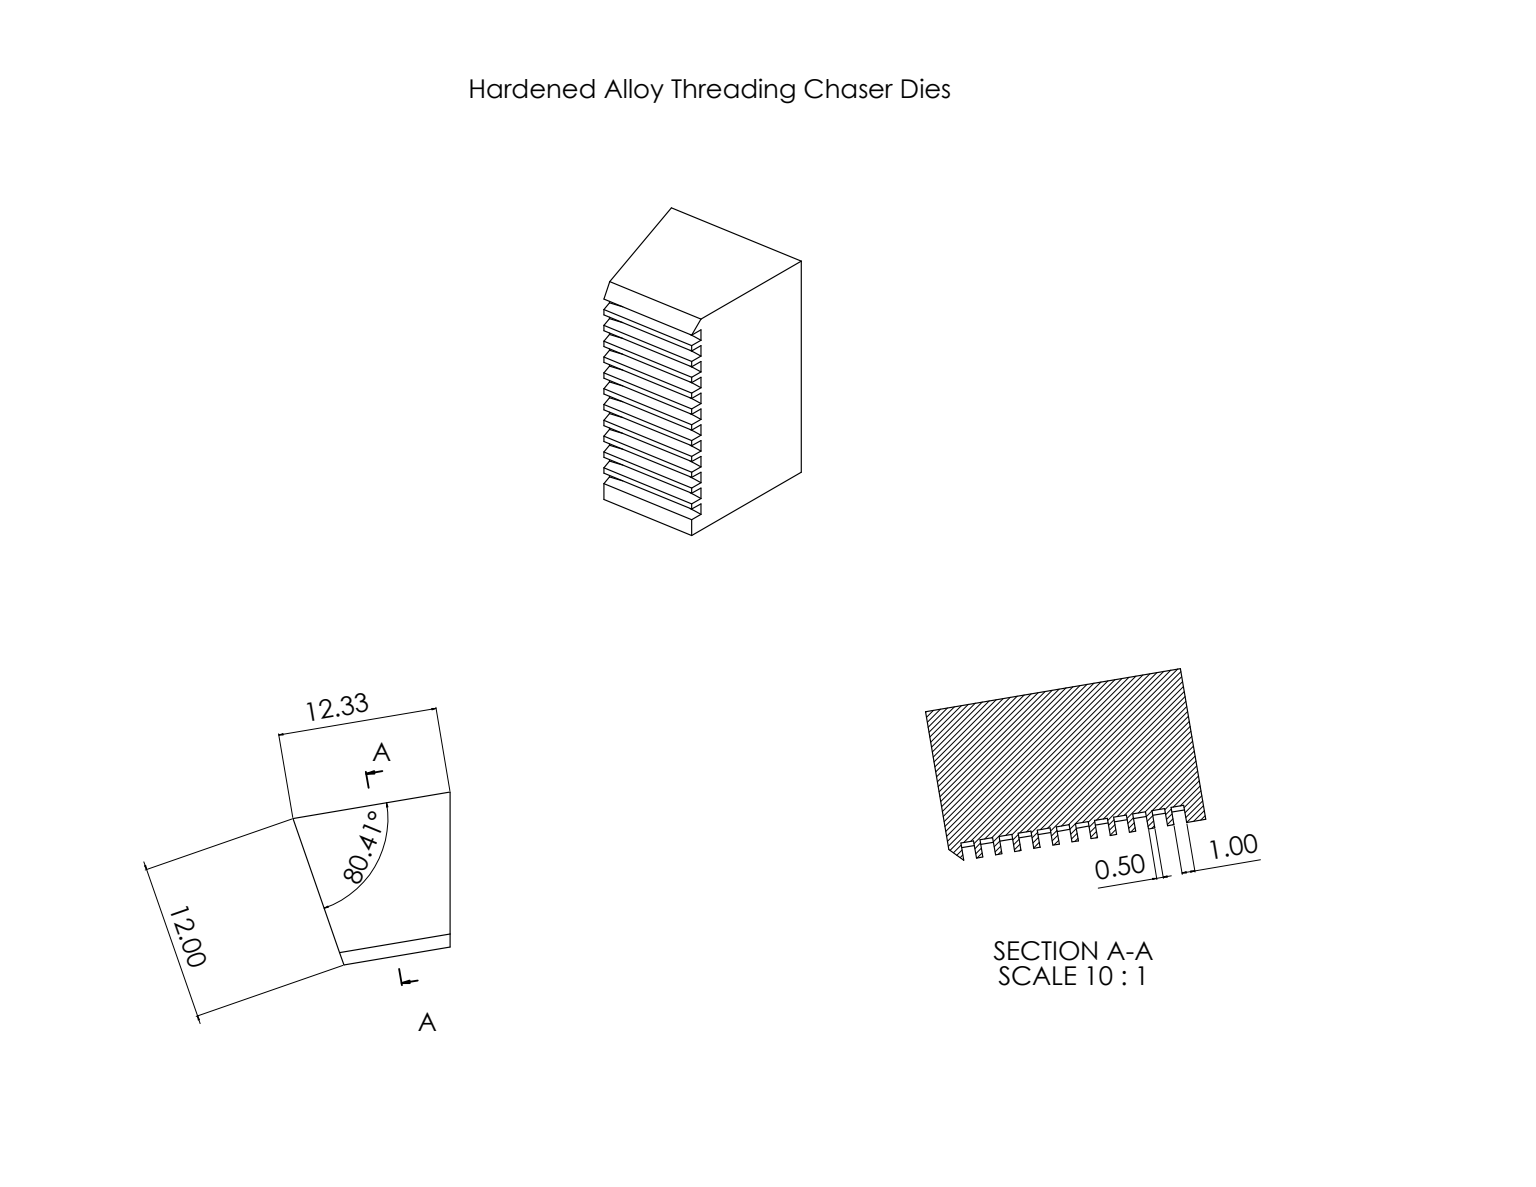
ISO-10303-21;
HEADER;
FILE_DESCRIPTION (('STEP AP214'),
    '1' );
FILE_NAME ('Hardened Alloy Threading Chaser Dies.step',
    '2026-10-19T14:05:14',
    ( '' ),
    ( '' ),
    'SwSTEP 2.0',
    'SolidWorks 2025',
    '' );
FILE_SCHEMA (( 'AUTOMOTIVE_DESIGN' ));
ENDSEC;

DATA;
#3=ORIENTED_EDGE ( 'NONE', *, *, #1774, .T. ) ;
#6=ORIENTED_EDGE ( 'NONE', *, *, #748, .T. ) ;
#8=LINE ( 'NONE', #7609, #8604 ) ;
#18=CARTESIAN_POINT ( 'NONE',  ( 1.030449557444946671E-26, 53.50000000000031264, -26.00000000000004974 ) ) ;
#24=ORIENTED_EDGE ( 'NONE', *, *, #464, .F. ) ;
#25=PRODUCT_DEFINITION_CONTEXT ( 'detailed design', #5808, 'design' ) ;
#30=FACE_OUTER_BOUND ( 'NONE', #6374, .T. ) ;
#38=CARTESIAN_POINT ( 'NONE',  ( 1.084683744678891232E-26, 59.63872771225970837, -25.64778813235487220 ) ) ;
#47=VECTOR ( 'NONE', #1280, 1000.000000000000000 ) ;
#49=VERTEX_POINT ( 'NONE', #7520 ) ;
#65=EDGE_LOOP ( 'NONE', ( #1698, #9286, #7170, #5423 ) ) ;
#70=CARTESIAN_POINT ( 'NONE',  ( 0.000000000000000000, 0.000000000000000000, 0.000000000000000000 ) ) ;
#75=DIRECTION ( 'NONE',  ( -1.735493991486225972E-29, 6.508102468073347395E-30, 1.000000000000000000 ) ) ;
#77=VERTEX_POINT ( 'NONE', #3810 ) ;
#83=CARTESIAN_POINT ( 'NONE',  ( 0.000000000000000000, 0.000000000000000000, 0.000000000000000000 ) ) ;
#90=AXIS2_PLACEMENT_3D ( 'NONE', #5171, #7481, #672 ) ;
#100=ORIENTED_EDGE ( 'NONE', *, *, #2687, .F. ) ;
#103=VECTOR ( 'NONE', #6274, 1000.000000000000341 ) ;
#104=CIRCLE ( 'NONE', #7815, 26.00000000000012790 ) ;
#107=EDGE_CURVE ( 'NONE', #2537, #9428, #3759, .T. ) ;
#110=CARTESIAN_POINT ( 'NONE',  ( 8.948640893600852668E-27, 42.50000000000020606, -25.00000000000000000 ) ) ;
#111=ORIENTED_EDGE ( 'NONE', *, *, #684, .T. ) ;
#114=ORIENTED_EDGE ( 'NONE', *, *, #8852, .F. ) ;
#117=AXIS2_PLACEMENT_3D ( 'NONE', #7294, #7143, #4982 ) ;
#119=CARTESIAN_POINT ( 'NONE',  ( -8.216777476527294510, 42.50000000000020606, -23.61111111111107519 ) ) ;
#125=CIRCLE ( 'NONE', #905, 26.00000000000000355 ) ;
#145=LINE ( 'NONE', #38, #7530 ) ;
#146=LINE ( 'NONE', #3335, #665 ) ;
#147=( LENGTH_UNIT ( ) NAMED_UNIT ( * ) SI_UNIT ( .MILLI., .METRE. ) );
#149=FACE_OUTER_BOUND ( 'NONE', #9484, .T. ) ;
#150=ADVANCED_FACE ( 'NONE', ( #6740 ), #686, .F. ) ;
#154=DIRECTION ( 'NONE',  ( 0.9860132971832693549, 1.788557213313974126E-28, -0.1666666666666657970 ) ) ;
#158=CARTESIAN_POINT ( 'NONE',  ( -8.216777476527294510, 50.00000000000032685, -23.61111111111111427 ) ) ;
#159=ORIENTED_EDGE ( 'NONE', *, *, #5056, .F. ) ;
#163=EDGE_CURVE ( 'NONE', #7794, #4048, #3844, .T. ) ;
#164=ADVANCED_FACE ( 'NONE', ( #5228 ), #5133, .F. ) ;
#185=VERTEX_POINT ( 'NONE', #9279 ) ;
#188=( GEOMETRIC_REPRESENTATION_CONTEXT ( 3 ) GLOBAL_UNCERTAINTY_ASSIGNED_CONTEXT ( ( #1496 ) ) GLOBAL_UNIT_ASSIGNED_CONTEXT ( ( #3676, #5943, #2174 ) ) REPRESENTATION_CONTEXT ( 'NONE', 'WORKASPACE' ) );
#195=ORIENTED_EDGE ( 'NONE', *, *, #1181, .F. ) ;
#214=CARTESIAN_POINT ( 'NONE',  ( 8.948640893600852668E-27, 42.50000000000020606, -25.00000000000000000 ) ) ;
#217=ADVANCED_FACE ( 'NONE', ( #8822 ), #7238, .F. ) ;
#226=EDGE_CURVE ( 'NONE', #987, #5419, #6349, .T. ) ;
#232=CARTESIAN_POINT ( 'NONE',  ( -8.545448575588375562, 56.00000000000030553, -24.55555555555558911 ) ) ;
#240=ORIENTED_EDGE ( 'NONE', *, *, #7837, .T. ) ;
#248=LINE ( 'NONE', #2485, #2906 ) ;
#250=AXIS2_PLACEMENT_3D ( 'NONE', #2833, #9708, #7388 ) ;
#255=EDGE_CURVE ( 'NONE', #1637, #4569, #2387, .T. ) ;
#260=DIRECTION ( 'NONE',  ( -1.735493991486225972E-29, 6.508102468073347395E-30, 1.000000000000000000 ) ) ;
#265=CARTESIAN_POINT ( 'NONE',  ( -8.216777476527294510, 56.50000000000029843, -23.61111111111111427 ) ) ;
#269=VERTEX_POINT ( 'NONE', #3889 ) ;
#274=VECTOR ( 'NONE', #1912, 1000.000000000000341 ) ;
#284=CARTESIAN_POINT ( 'NONE',  ( 9.318419442923201951E-27, 47.00000000000034106, -25.00000000000000000 ) ) ;
#302=CARTESIAN_POINT ( 'NONE',  ( 9.762153702110021092E-27, 45.50000000000019185, -25.00000000000000000 ) ) ;
#309=CARTESIAN_POINT ( 'NONE',  ( 9.219811829770575476E-27, 48.50000000000033396, -26.00000000000011369 ) ) ;
#318=ORIENTED_EDGE ( 'NONE', *, *, #9442, .F. ) ;
#319=AXIS2_PLACEMENT_3D ( 'NONE', #6643, #8980, #9669 ) ;
#321=ORIENTED_EDGE ( 'NONE', *, *, #7835, .T. ) ;
#336=VECTOR ( 'NONE', #2888, 1000.000000000000000 ) ;
#346=AXIS2_PLACEMENT_3D ( 'NONE', #4083, #2634, #9223 ) ;
#358=AXIS2_PLACEMENT_3D ( 'NONE', #6746, #9141, #8245 ) ;
#364=ORIENTED_EDGE ( 'NONE', *, *, #965, .F. ) ;
#369=ORIENTED_EDGE ( 'NONE', *, *, #9442, .T. ) ;
#375=CARTESIAN_POINT ( 'NONE',  ( 1.203012880462043003E-26, 59.00000000000029843, -25.00000000000000000 ) ) ;
#379=EDGE_LOOP ( 'NONE', ( #2512, #3295, #4858, #1225 ) ) ;
#382=FACE_OUTER_BOUND ( 'NONE', #3255, .T. ) ;
#393=DIRECTION ( 'NONE',  ( 1.735493991486225972E-29, -6.508102468073347395E-30, -1.000000000000000000 ) ) ;
#395=PLANE ( 'NONE',  #2897 ) ;
#408=ORIENTED_EDGE ( 'NONE', *, *, #8224, .T. ) ;
#445=FACE_OUTER_BOUND ( 'NONE', #6404, .T. ) ;
#451=DIRECTION ( 'NONE',  ( -1.735493991486225972E-29, 6.508102468073347395E-30, 1.000000000000000000 ) ) ;
#463=EDGE_CURVE ( 'NONE', #6976, #7794, #626, .T. ) ;
#464=EDGE_CURVE ( 'NONE', #7542, #9099, #8278, .T. ) ;
#467=LINE ( 'NONE', #608, #6068 ) ;
#468=EDGE_CURVE ( 'NONE', #5208, #1296, #1199, .T. ) ;
#473=ORIENTED_EDGE ( 'NONE', *, *, #8224, .F. ) ;
#478=VERTEX_POINT ( 'NONE', #8225 ) ;
#481=ORIENTED_EDGE ( 'NONE', *, *, #7790, .F. ) ;
#482=CARTESIAN_POINT ( 'NONE',  ( -8.216777476527274970, 48.50000000000033396, -23.61111111111111427 ) ) ;
#488=CARTESIAN_POINT ( 'NONE',  ( 1.555535097482682654E-26, 78.08723716182652197, -25.00000000000000000 ) ) ;
#495=PLANE ( 'NONE',  #7443 ) ;
#496=DIRECTION ( 'NONE',  ( -0.9860132971832694659, -1.788557213313974350E-28, 0.1666666666666658247 ) ) ;
#501=ORIENTED_EDGE ( 'NONE', *, *, #2623, .T. ) ;
#517=VERTEX_POINT ( 'NONE', #5126 ) ;
#518=EDGE_LOOP ( 'NONE', ( #1786, #1861, #2119, #8803 ) ) ;
#524=ADVANCED_FACE ( 'NONE', ( #4341 ), #7345, .F. ) ;
#530=ORIENTED_EDGE ( 'NONE', *, *, #3207, .T. ) ;
#532=VECTOR ( 'NONE', #9646, 1000.000000000000341 ) ;
#534=LINE ( 'NONE', #2734, #9462 ) ;
#544=CARTESIAN_POINT ( 'NONE',  ( 5.423418723394456162E-28, -2.066522830327504070E-28, -26.00000000000000355 ) ) ;
#545=DIRECTION ( 'NONE',  ( 1.735493991486223450E-29, 0.000000000000000000, -1.000000000000000000 ) ) ;
#553=EDGE_CURVE ( 'NONE', #1486, #2396, #9731, .T. ) ;
#554=ORIENTED_EDGE ( 'NONE', *, *, #4928, .F. ) ;
#571=AXIS2_PLACEMENT_3D ( 'NONE', #1883, #7968, #2471 ) ;
#574=EDGE_CURVE ( 'NONE', #9611, #2873, #3443, .T. ) ;
#578=CARTESIAN_POINT ( 'NONE',  ( 7.913260955498274673E-27, 41.50000000000020606, -26.00000000000017408 ) ) ;
#580=DIRECTION ( 'NONE',  ( -1.820952055660014662E-28, -1.000000000000000000, -7.038118388768679669E-30 ) ) ;
#586=EDGE_CURVE ( 'NONE', #9099, #2192, #627, .T. ) ;
#599=CARTESIAN_POINT ( 'NONE',  ( -8.216777476527274970, 47.50000000000033396, -23.61111111111111427 ) ) ;
#608=CARTESIAN_POINT ( 'NONE',  ( 1.040310318760209318E-26, 47.00000000000034106, -37.00000000000000711 ) ) ;
#611=ORIENTED_EDGE ( 'NONE', *, *, #2805, .F. ) ;
#615=CARTESIAN_POINT ( 'NONE',  ( 9.860761315262647568E-27, 50.00000000000032685, -24.09806918451531033 ) ) ;
#616=CARTESIAN_POINT ( 'NONE',  ( -8.216777476527274970, 78.08723716182652197, -23.61111111111111427 ) ) ;
#626=LINE ( 'NONE', #5323, #2764 ) ;
#627=LINE ( 'NONE', #6495, #5483 ) ;
#628=DIRECTION ( 'NONE',  ( 1.735493991486225692E-29, 0.000000000000000000, -1.000000000000000000 ) ) ;
#631=VECTOR ( 'NONE', #3107, 1000.000000000000000 ) ;
#643=ORIENTED_EDGE ( 'NONE', *, *, #1715, .F. ) ;
#647=DIRECTION ( 'NONE',  ( 1.735493991486224571E-29, 0.000000000000000000, -1.000000000000000000 ) ) ;
#648=CARTESIAN_POINT ( 'NONE',  ( 9.762153702110021092E-27, 45.50000000000019185, -37.00000000000000711 ) ) ;
#649=EDGE_CURVE ( 'NONE', #2857, #6423, #145, .T. ) ;
#652=AXIS2_PLACEMENT_3D ( 'NONE', #8214, #4323, #7326 ) ;
#653=AXIS2_PLACEMENT_3D ( 'NONE', #663, #4395, #7445 ) ;
#659=DIRECTION ( 'NONE',  ( -1.820952055660014662E-28, -1.000000000000000000, -7.038118388768679669E-30 ) ) ;
#660=ORIENTED_EDGE ( 'NONE', *, *, #3351, .F. ) ;
#663=CARTESIAN_POINT ( 'NONE',  ( 1.555535097482682654E-26, 78.08723716182652197, -25.00000000000000000 ) ) ;
#665=VECTOR ( 'NONE', #3132, 1000.000000000000000 ) ;
#667=VERTEX_POINT ( 'NONE', #3684 ) ;
#672=DIRECTION ( 'NONE',  ( 1.735493991486225411E-29, 0.000000000000000000, -1.000000000000000000 ) ) ;
#677=LINE ( 'NONE', #6683, #1670 ) ;
#683=VECTOR ( 'NONE', #8096, 1000.000000000000000 ) ;
#684=EDGE_CURVE ( 'NONE', #7011, #7381, #677, .T. ) ;
#686=PLANE ( 'NONE',  #5828 ) ;
#689=LINE ( 'NONE', #2993, #4805 ) ;
#698=ORIENTED_EDGE ( 'NONE', *, *, #2685, .T. ) ;
#701=CARTESIAN_POINT ( 'NONE',  ( 1.002605232869780806E-26, 55.00000000000030553, 3.131562089573645497E-28 ) ) ;
#706=ORIENTED_EDGE ( 'NONE', *, *, #9278, .T. ) ;
#708=AXIS2_PLACEMENT_3D ( 'NONE', #7091, #1077, #2399 ) ;
#710=EDGE_CURVE ( 'NONE', #1005, #1238, #6143, .T. ) ;
#713=CARTESIAN_POINT ( 'NONE',  ( -8.545448575588398654, 44.00000000000019895, -24.55555555555570990 ) ) ;
#721=CIRCLE ( 'NONE', #90, 26.00000000000004974 ) ;
#724=CARTESIAN_POINT ( 'NONE',  ( 8.726773764007443097E-27, 41.50000000000020606, -37.00000000000000711 ) ) ;
#729=ORIENTED_EDGE ( 'NONE', *, *, #5227, .T. ) ;
#733=CARTESIAN_POINT ( 'NONE',  ( -8.216777476527274970, 78.08723716182652197, -23.61111111111111427 ) ) ;
#738=CYLINDRICAL_SURFACE ( 'NONE', #9058, 26.00000000000002132 ) ;
#746=CARTESIAN_POINT ( 'NONE',  ( 0.000000000000000000, 0.000000000000000000, 0.000000000000000000 ) ) ;
#748=EDGE_CURVE ( 'NONE', #1486, #8507, #3031, .T. ) ;
#760=EDGE_CURVE ( 'NONE', #4270, #9740, #8481, .T. ) ;
#762=ADVANCED_FACE ( 'NONE', ( #4778 ), #1708, .F. ) ;
#770=ADVANCED_FACE ( 'NONE', ( #7031 ), #5661, .F. ) ;
#771=ADVANCED_FACE ( 'NONE', ( #8525 ), #8673, .F. ) ;
#773=CARTESIAN_POINT ( 'NONE',  ( -8.216777476527274970, 78.08723716182652197, -23.61111111111111427 ) ) ;
#777=CARTESIAN_POINT ( 'NONE',  ( 8.577746286997626155E-27, 47.00000000000034106, 1.660151612061797305E-28 ) ) ;
#781=ORIENTED_EDGE ( 'NONE', *, *, #7457, .T. ) ;
#785=DIRECTION ( 'NONE',  ( -1.820952055660014662E-28, -1.000000000000000000, -7.038118388768679669E-30 ) ) ;
#793=ADVANCED_FACE ( 'NONE', ( #1018 ), #6391, .T. ) ;
#798=ORIENTED_EDGE ( 'NONE', *, *, #1487, .T. ) ;
#821=EDGE_CURVE ( 'NONE', #9092, #667, #3230, .T. ) ;
#829=DIRECTION ( 'NONE',  ( -1.820952055660014662E-28, -1.000000000000000000, -7.038118388768679669E-30 ) ) ;
#854=DIRECTION ( 'NONE',  ( -1.820952055660014662E-28, -1.000000000000000000, -7.038118388768679669E-30 ) ) ;
#883=DIRECTION ( 'NONE',  ( -0.3286710990610922090, -6.289316826390952918E-29, -0.9444444444444435316 ) ) ;
#890=EDGE_CURVE ( 'NONE', #9115, #5960, #5703, .T. ) ;
#892=VECTOR ( 'NONE', #8543, 1000.000000000000341 ) ;
#905=AXIS2_PLACEMENT_3D ( 'NONE', #6737, #5223, #7491 ) ;
#906=LINE ( 'NONE', #1540, #8759 ) ;
#918=PLANE ( 'NONE',  #6689 ) ;
#923=DIRECTION ( 'NONE',  ( 1.820952055660014662E-28, 1.000000000000000000, -6.508102468073347395E-30 ) ) ;
#929=LINE ( 'NONE', #1025, #9706 ) ;
#930=EDGE_CURVE ( 'NONE', #7030, #7610, #9528, .T. ) ;
#937=EDGE_CURVE ( 'NONE', #1495, #1081, #5017, .T. ) ;
#945=ORIENTED_EDGE ( 'NONE', *, *, #8555, .F. ) ;
#947=DIRECTION ( 'NONE',  ( 1.735493991486225692E-29, -6.508102468073347395E-30, -1.000000000000000000 ) ) ;
#955=VECTOR ( 'NONE', #1121, 1000.000000000000000 ) ;
#956=EDGE_LOOP ( 'NONE', ( #1913, #7125, #1447, #1645 ) ) ;
#959=ORIENTED_EDGE ( 'NONE', *, *, #6232, .F. ) ;
#965=EDGE_CURVE ( 'NONE', #2396, #1296, #7185, .T. ) ;
#973=DIRECTION ( 'NONE',  ( -1.820952055660014662E-28, -1.000000000000000000, -7.038118388768679669E-30 ) ) ;
#987=VERTEX_POINT ( 'NONE', #5846 ) ;
#990=CARTESIAN_POINT ( 'NONE',  ( -8.216777476527294510, 53.00000000000031974, -23.61111111111111427 ) ) ;
#994=CARTESIAN_POINT ( 'NONE',  ( -8.550110809860612449, 60.00000000000029843, -24.56895259980339929 ) ) ;
#997=DIRECTION ( 'NONE',  ( -1.820952055660014662E-28, -1.000000000000000000, -7.038118388768679669E-30 ) ) ;
#1000=EDGE_CURVE ( 'NONE', #7794, #6031, #8346, .T. ) ;
#1005=VERTEX_POINT ( 'NONE', #7661 ) ;
#1008=VERTEX_POINT ( 'NONE', #8884 ) ;
#1015=AXIS2_PLACEMENT_3D ( 'NONE', #5064, #4381, #9466 ) ;
#1018=FACE_OUTER_BOUND ( 'NONE', #7000, .T. ) ;
#1025=CARTESIAN_POINT ( 'NONE',  ( -8.216777476527274970, 78.08723716182652197, -23.61111111111111427 ) ) ;
#1027=LINE ( 'NONE', #9185, #3047 ) ;
#1032=ORIENTED_EDGE ( 'NONE', *, *, #4563, .F. ) ;
#1033=AXIS2_PLACEMENT_3D ( 'NONE', #7668, #8998, #6121 ) ;
#1038=VECTOR ( 'NONE', #8996, 1000.000000000000341 ) ;
#1043=ORIENTED_EDGE ( 'NONE', *, *, #3461, .F. ) ;
#1044=DIRECTION ( 'NONE',  ( -1.820952055660014662E-28, -1.000000000000000000, -7.038118388768679669E-30 ) ) ;
#1056=EDGE_LOOP ( 'NONE', ( #554, #4946, #5055, #1032 ) ) ;
#1077=DIRECTION ( 'NONE',  ( -1.820459017594251978E-28, -1.000000000000000000, 6.508102468073347395E-30 ) ) ;
#1081=VERTEX_POINT ( 'NONE', #1716 ) ;
#1082=CARTESIAN_POINT ( 'NONE',  ( -8.216777476527274970, 47.00000000000034106, -23.61111111111107519 ) ) ;
#1102=VECTOR ( 'NONE', #3641, 1000.000000000000000 ) ;
#1107=CARTESIAN_POINT ( 'NONE',  ( -4.275055404930308001, 60.00000000000029843, -25.29156885273883049 ) ) ;
#1108=EDGE_CURVE ( 'NONE', #667, #2443, #4931, .T. ) ;
#1117=DIRECTION ( 'NONE',  ( -1.820952055660014662E-28, -1.000000000000000000, -7.038118388768679669E-30 ) ) ;
#1120=CARTESIAN_POINT ( 'NONE',  ( -8.216777476527294510, 59.00000000000029843, -23.61111111111111427 ) ) ;
#1121=DIRECTION ( 'NONE',  ( 1.735493991486225972E-29, -6.508102468073347395E-30, -1.000000000000000000 ) ) ;
#1127=ADVANCED_FACE ( 'NONE', ( #5189 ), #5237, .F. ) ;
#1132=DIRECTION ( 'NONE',  ( -1.820952055660014662E-28, -1.000000000000000000, 6.508102468073347395E-30 ) ) ;
#1146=DIRECTION ( 'NONE',  ( -1.820952055660014662E-28, -1.000000000000000000, -7.038118388768679669E-30 ) ) ;
#1150=ORIENTED_EDGE ( 'NONE', *, *, #9390, .T. ) ;
#1153=ORIENTED_EDGE ( 'NONE', *, *, #2248, .F. ) ;
#1154=CARTESIAN_POINT ( 'NONE',  ( -8.216777476527274970, 78.08723716182652197, -23.61111111111111427 ) ) ;
#1161=DIRECTION ( 'NONE',  ( 1.820952055660014662E-28, 1.000000000000000000, 7.038118388768679669E-30 ) ) ;
#1164=ORIENTED_EDGE ( 'NONE', *, *, #2925, .F. ) ;
#1174=VECTOR ( 'NONE', #5910, 1000.000000000000341 ) ;
#1177=CARTESIAN_POINT ( 'NONE',  ( 7.824319130992849937E-27, 43.00000000000019895, 2.858080037470658006E-28 ) ) ;
#1178=PLANE ( 'NONE',  #117 ) ;
#1181=EDGE_CURVE ( 'NONE', #2714, #269, #5546, .T. ) ;
#1182=CARTESIAN_POINT ( 'NONE',  ( 9.219811829770575476E-27, 40.00000000000014921, -37.00000000000000711 ) ) ;
#1188=VECTOR ( 'NONE', #5184, 1000.000000000000000 ) ;
#1197=CARTESIAN_POINT ( 'NONE',  ( -12.16083066526040213, 78.08723716182652197, -34.94444444444459918 ) ) ;
#1199=CIRCLE ( 'NONE', #7202, 26.00000000000017408 ) ;
#1204=LINE ( 'NONE', #4953, #2126 ) ;
#1207=CARTESIAN_POINT ( 'NONE',  ( 1.138917931912835794E-26, 56.00000000000030553, -25.00000000000000000 ) ) ;
#1212=DIRECTION ( 'NONE',  ( -1.820952055660014662E-28, -1.000000000000000000, -7.038118388768679669E-30 ) ) ;
#1225=ORIENTED_EDGE ( 'NONE', *, *, #7891, .F. ) ;
#1230=CARTESIAN_POINT ( 'NONE',  ( 1.000867273499158728E-26, 44.50000000000019185, -37.00000000000000711 ) ) ;
#1231=DIRECTION ( 'NONE',  ( -0.1666666666666658525, -3.897465909857536228E-29, -0.9860132971832695770 ) ) ;
#1238=VERTEX_POINT ( 'NONE', #8812 ) ;
#1253=EDGE_LOOP ( 'NONE', ( #2425, #643, #8630, #4172 ) ) ;
#1270=ADVANCED_BREP_SHAPE_REPRESENTATION ( '', ( #9647, #6314 ), #188 ) ;
#1271=ADVANCED_FACE ( 'NONE', ( #4421 ), #3672, .F. ) ;
#1275=DIRECTION ( 'NONE',  ( 1.735493991486225972E-29, -6.508102468073347395E-30, -1.000000000000000000 ) ) ;
#1280=DIRECTION ( 'NONE',  ( -1.820952055660014662E-28, -1.000000000000000000, -7.038118388768679669E-30 ) ) ;
#1281=VECTOR ( 'NONE', #2735, 1000.000000000000000 ) ;
#1290=DIRECTION ( 'NONE',  ( -0.9860132971832693549, -1.788557213313974126E-28, 0.1666666666666657970 ) ) ;
#1291=DIRECTION ( 'NONE',  ( 1.735493991486225972E-29, -6.508102468073347395E-30, -1.000000000000000000 ) ) ;
#1293=VECTOR ( 'NONE', #1382, 1000.000000000000000 ) ;
#1296=VERTEX_POINT ( 'NONE', #578 ) ;
#1298=ORIENTED_EDGE ( 'NONE', *, *, #4743, .F. ) ;
#1300=ORIENTED_EDGE ( 'NONE', *, *, #4920, .F. ) ;
#1304=LINE ( 'NONE', #8958, #5871 ) ;
#1308=ORIENTED_EDGE ( 'NONE', *, *, #6948, .F. ) ;
#1312=DIRECTION ( 'NONE',  ( -1.735493991486225972E-29, 6.508102468073347395E-30, 1.000000000000000000 ) ) ;
#1314=CARTESIAN_POINT ( 'NONE',  ( -8.545448575588366680, 59.00000000000029843, -24.55555555555556424 ) ) ;
#1325=DIRECTION ( 'NONE',  ( -1.000000000000000000, -1.821691612758658688E-28, -1.735493991486225972E-29 ) ) ;
#1326=DIRECTION ( 'NONE',  ( 1.820952055660014662E-28, 1.000000000000000000, 7.038118388768679669E-30 ) ) ;
#1329=ORIENTED_EDGE ( 'NONE', *, *, #2926, .F. ) ;
#1336=DIRECTION ( 'NONE',  ( -1.820952055660014662E-28, -1.000000000000000000, -7.038118388768679669E-30 ) ) ;
#1340=AXIS2_PLACEMENT_3D ( 'NONE', #8032, #8636, #2686 ) ;
#1346=FACE_OUTER_BOUND ( 'NONE', #518, .T. ) ;
#1347=ORIENTED_EDGE ( 'NONE', *, *, #1633, .T. ) ;
#1359=DIRECTION ( 'NONE',  ( 1.735493991486224571E-29, 0.000000000000000000, -1.000000000000000000 ) ) ;
#1378=ORIENTED_EDGE ( 'NONE', *, *, #5490, .F. ) ;
#1382=DIRECTION ( 'NONE',  ( -1.820952055660014662E-28, -1.000000000000000000, -7.038118388768679669E-30 ) ) ;
#1393=CARTESIAN_POINT ( 'NONE',  ( 5.423418723394456162E-28, -2.066522830327504070E-28, -26.00000000000009592 ) ) ;
#1397=DIRECTION ( 'NONE',  ( 1.735493991486227373E-29, 0.000000000000000000, -1.000000000000000000 ) ) ;
#1407=EDGE_CURVE ( 'NONE', #6987, #2912, #2825, .T. ) ;
#1411=DIRECTION ( 'NONE',  ( 1.735493991486225972E-29, -6.508102468073347395E-30, -1.000000000000000000 ) ) ;
#1423=ORIENTED_EDGE ( 'NONE', *, *, #5719, .T. ) ;
#1447=ORIENTED_EDGE ( 'NONE', *, *, #9031, .T. ) ;
#1451=CYLINDRICAL_SURFACE ( 'NONE', #9001, 26.00000000000000355 ) ;
#1455=LINE ( 'NONE', #1868, #2834 ) ;
#1457=DIRECTION ( 'NONE',  ( -1.820952055660014662E-28, -1.000000000000000000, -7.038118388768679669E-30 ) ) ;
#1482=CARTESIAN_POINT ( 'NONE',  ( -8.216777476527294510, 58.00000000000029132, -23.61111111111107519 ) ) ;
#1483=SHAPE_REPRESENTATION ( 'Hardened Alloy Threading Chaser Dies', ( #6314 ), #188 ) ;
#1486=VERTEX_POINT ( 'NONE', #5357 ) ;
#1487=EDGE_CURVE ( 'NONE', #2912, #3082, #1601, .T. ) ;
#1489=EDGE_CURVE ( 'NONE', #3682, #6660, #4668, .T. ) ;
#1495=VERTEX_POINT ( 'NONE', #5593 ) ;
#1496=UNCERTAINTY_MEASURE_WITH_UNIT (LENGTH_MEASURE( 1.000000000000000082E-05 ), #3676, 'distance_accuracy_value', 'NONE');
#1497=CIRCLE ( 'NONE', #2113, 26.00000000000008171 ) ;
#1512=DIRECTION ( 'NONE',  ( 1.735493991486228214E-29, 0.000000000000000000, -1.000000000000000000 ) ) ;
#1525=LINE ( 'NONE', #6847, #5872 ) ;
#1535=ORIENTED_EDGE ( 'NONE', *, *, #7835, .F. ) ;
#1540=CARTESIAN_POINT ( 'NONE',  ( -12.16083066526040213, 60.00000000000029843, -34.94444444444452103 ) ) ;
#1549=EDGE_CURVE ( 'NONE', #5397, #3824, #7873, .T. ) ;
#1556=LINE ( 'NONE', #7309, #3942 ) ;
#1562=ORIENTED_EDGE ( 'NONE', *, *, #1489, .F. ) ;
#1565=LINE ( 'NONE', #9024, #4826 ) ;
#1581=ORIENTED_EDGE ( 'NONE', *, *, #7790, .T. ) ;
#1583=VECTOR ( 'NONE', #8478, 1000.000000000000000 ) ;
#1601=LINE ( 'NONE', #6873, #3070 ) ;
#1604=AXIS2_PLACEMENT_3D ( 'NONE', #7690, #923, #3935 ) ;
#1605=DIRECTION ( 'NONE',  ( -1.820952055660014662E-28, -1.000000000000000000, 6.508102468073347395E-30 ) ) ;
#1620=ORIENTED_EDGE ( 'NONE', *, *, #468, .T. ) ;
#1621=PLANE ( 'NONE',  #6048 ) ;
#1633=EDGE_CURVE ( 'NONE', #2537, #7542, #1204, .T. ) ;
#1637=VERTEX_POINT ( 'NONE', #2023 ) ;
#1642=AXIS2_PLACEMENT_3D ( 'NONE', #3342, #6891, #6351 ) ;
#1645=ORIENTED_EDGE ( 'NONE', *, *, #821, .F. ) ;
#1654=CARTESIAN_POINT ( 'NONE',  ( 8.455602827837720289E-27, 41.50000000000020606, -25.00000000000000000 ) ) ;
#1655=VECTOR ( 'NONE', #8004, 1000.000000000000000 ) ;
#1656=ADVANCED_FACE ( 'NONE', ( #9542 ), #4222, .F. ) ;
#1666=DIRECTION ( 'NONE',  ( -0.1666666666666658525, -3.897465909857536228E-29, -0.9860132971832695770 ) ) ;
#1670=VECTOR ( 'NONE', #1457, 1000.000000000000000 ) ;
#1672=EDGE_CURVE ( 'NONE', #7720, #49, #467, .T. ) ;
#1675=LINE ( 'NONE', #1813, #6043 ) ;
#1679=LINE ( 'NONE', #2542, #7677 ) ;
#1681=LINE ( 'NONE', #6112, #2535 ) ;
#1683=DIRECTION ( 'NONE',  ( -1.820952055660014662E-28, -1.000000000000000000, -7.038118388768679669E-30 ) ) ;
#1690=ORIENTED_EDGE ( 'NONE', *, *, #3745, .T. ) ;
#1693=DIRECTION ( 'NONE',  ( 1.735493991486225972E-29, -6.508102468073347395E-30, -1.000000000000000000 ) ) ;
#1698=ORIENTED_EDGE ( 'NONE', *, *, #3775, .F. ) ;
#1706=ORIENTED_EDGE ( 'NONE', *, *, #9014, .T. ) ;
#1708=PLANE ( 'NONE',  #346 ) ;
#1714=EDGE_CURVE ( 'NONE', #6660, #7461, #5135, .T. ) ;
#1715=EDGE_CURVE ( 'NONE', #5638, #8408, #6614, .T. ) ;
#1716=CARTESIAN_POINT ( 'NONE',  ( 9.860761315262647568E-27, 49.00000000000032685, -25.00000000000000000 ) ) ;
#1717=DIRECTION ( 'NONE',  ( 1.735493991486225972E-29, -6.508102468073347395E-30, -1.000000000000000000 ) ) ;
#1729=VECTOR ( 'NONE', #3773, 1000.000000000000000 ) ;
#1746=ORIENTED_EDGE ( 'NONE', *, *, #7023, .F. ) ;
#1751=CARTESIAN_POINT ( 'NONE',  ( -8.429686713947083021, 59.63872771225970837, -24.22291101389071244 ) ) ;
#1753=DIRECTION ( 'NONE',  ( 0.3286710990610922090, 6.289316826390952918E-29, 0.9444444444444435316 ) ) ;
#1756=CARTESIAN_POINT ( 'NONE',  ( -8.545448575588402207, 41.50000000000020606, -24.55555555555572411 ) ) ;
#1774=EDGE_CURVE ( 'NONE', #987, #8311, #7660, .T. ) ;
#1777=CARTESIAN_POINT ( 'NONE',  ( 8.653435754032105718E-27, 47.50000000000033396, 3.062228611575705006E-28 ) ) ;
#1780=EDGE_CURVE ( 'NONE', #6156, #6996, #5343, .T. ) ;
#1786=ORIENTED_EDGE ( 'NONE', *, *, #5350, .F. ) ;
#1788=EDGE_CURVE ( 'NONE', #9115, #9126, #3886, .T. ) ;
#1794=CARTESIAN_POINT ( 'NONE',  ( 8.825381377160069573E-27, 47.00000000000034106, -24.09806918451533875 ) ) ;
#1797=EDGE_LOOP ( 'NONE', ( #8586, #5702, #530, #3613 ) ) ;
#1799=VECTOR ( 'NONE', #1312, 1000.000000000000000 ) ;
#1800=ORIENTED_EDGE ( 'NONE', *, *, #4335, .T. ) ;
#1802=LINE ( 'NONE', #1393, #4679 ) ;
#1803=CARTESIAN_POINT ( 'NONE',  ( 1.555535097482682654E-26, 78.08723716182652197, -25.00000000000000000 ) ) ;
#1813=CARTESIAN_POINT ( 'NONE',  ( -8.216777476527294510, 53.00000000000031974, -23.61111111111111427 ) ) ;
#1819=ORIENTED_EDGE ( 'NONE', *, *, #7225, .T. ) ;
#1827=CARTESIAN_POINT ( 'NONE',  ( -8.216777476527274970, 78.08723716182652197, -23.61111111111111427 ) ) ;
#1829=ORIENTED_EDGE ( 'NONE', *, *, #5990, .T. ) ;
#1833=ORIENTED_EDGE ( 'NONE', *, *, #4920, .T. ) ;
#1837=ADVANCED_FACE ( 'NONE', ( #7614 ), #6073, .F. ) ;
#1839=ORIENTED_EDGE ( 'NONE', *, *, #2828, .F. ) ;
#1843=FACE_OUTER_BOUND ( 'NONE', #379, .T. ) ;
#1844=ORIENTED_EDGE ( 'NONE', *, *, #7508, .T. ) ;
#1848=EDGE_CURVE ( 'NONE', #7524, #9587, #7667, .T. ) ;
#1850=ORIENTED_EDGE ( 'NONE', *, *, #1714, .T. ) ;
#1852=ORIENTED_EDGE ( 'NONE', *, *, #3562, .T. ) ;
#1853=DIRECTION ( 'NONE',  ( 1.735493991486225972E-29, -6.508102468073347395E-30, -1.000000000000000000 ) ) ;
#1858=CARTESIAN_POINT ( 'NONE',  ( 8.677469957431129860E-27, 43.00000000000019895, -37.00000000000000711 ) ) ;
#1859=ORIENTED_EDGE ( 'NONE', *, *, #4933, .F. ) ;
#1860=CARTESIAN_POINT ( 'NONE',  ( 8.406299021261407051E-27, 42.50000000000020606, -26.00000000000017408 ) ) ;
#1861=ORIENTED_EDGE ( 'NONE', *, *, #163, .F. ) ;
#1868=CARTESIAN_POINT ( 'NONE',  ( 1.084683744678891232E-26, 53.00000000000031974, -37.00000000000000711 ) ) ;
#1871=DIRECTION ( 'NONE',  ( -1.820952055660014662E-28, -1.000000000000000000, -7.038118388768679669E-30 ) ) ;
#1873=ORIENTED_EDGE ( 'NONE', *, *, #5227, .F. ) ;
#1883=CARTESIAN_POINT ( 'NONE',  ( 0.000000000000000000, 0.000000000000000000, 0.000000000000000000 ) ) ;
#1884=EDGE_LOOP ( 'NONE', ( #1300, #4459, #9241, #2938 ) ) ;
#1892=AXIS2_PLACEMENT_3D ( 'NONE', #5608, #4867, #4132 ) ;
#1895=ORIENTED_EDGE ( 'NONE', *, *, #3169, .F. ) ;
#1898=EDGE_CURVE ( 'NONE', #3824, #1931, #7048, .T. ) ;
#1904=CIRCLE ( 'NONE', #3160, 26.00000000000009592 ) ;
#1910=VERTEX_POINT ( 'NONE', #7864 ) ;
#1912=DIRECTION ( 'NONE',  ( -0.9860132971832693549, -1.788557213313974126E-28, 0.1666666666666657970 ) ) ;
#1913=ORIENTED_EDGE ( 'NONE', *, *, #3038, .F. ) ;
#1916=AXIS2_PLACEMENT_3D ( 'NONE', #3446, #4935, #5858 ) ;
#1929=ORIENTED_EDGE ( 'NONE', *, *, #1549, .T. ) ;
#1931=VERTEX_POINT ( 'NONE', #990 ) ;
#1939=CARTESIAN_POINT ( 'NONE',  ( 9.219811829770575476E-27, 40.00000000000014921, -37.00000000000000711 ) ) ;
#1953=ORIENTED_EDGE ( 'NONE', *, *, #8512, .F. ) ;
#1966=FACE_OUTER_BOUND ( 'NONE', #6966, .T. ) ;
#1978=EDGE_CURVE ( 'NONE', #3873, #5638, #6998, .T. ) ;
#1991=VECTOR ( 'NONE', #8240, 1000.000000000000000 ) ;
#1996=CARTESIAN_POINT ( 'NONE',  ( 8.948640893600852668E-27, 42.50000000000020606, -24.09806918451538849 ) ) ;
#2011=ORIENTED_EDGE ( 'NONE', *, *, #760, .T. ) ;
#2023=CARTESIAN_POINT ( 'NONE',  ( 8.455602827837720289E-27, 41.50000000000020606, -25.00000000000000000 ) ) ;
#2025=DIRECTION ( 'NONE',  ( -1.735493991486225972E-29, 6.508102468073347395E-30, 1.000000000000000000 ) ) ;
#2026=ORIENTED_EDGE ( 'NONE', *, *, #2441, .F. ) ;
#2027=CARTESIAN_POINT ( 'NONE',  ( 0.000000000000000000, 0.000000000000000000, 0.000000000000000000 ) ) ;
#2029=CARTESIAN_POINT ( 'NONE',  ( -8.216777476527274970, 78.08723716182652197, -23.61111111111111427 ) ) ;
#2033=AXIS2_PLACEMENT_3D ( 'NONE', #1803, #9225, #9178 ) ;
#2045=DIRECTION ( 'NONE',  ( -0.1666666666666658525, -3.897465909857536228E-29, -0.9860132971832695770 ) ) ;
#2049=PLANE ( 'NONE',  #6677 ) ;
#2050=ORIENTED_EDGE ( 'NONE', *, *, #3287, .T. ) ;
#2051=DIRECTION ( 'NONE',  ( -1.820952055660014662E-28, -1.000000000000000000, -7.038118388768679669E-30 ) ) ;
#2059=CARTESIAN_POINT ( 'NONE',  ( 1.094544505994153880E-26, 52.00000000000031974, -37.00000000000000711 ) ) ;
#2065=ORIENTED_EDGE ( 'NONE', *, *, #7997, .T. ) ;
#2068=VECTOR ( 'NONE', #997, 1000.000000000000000 ) ;
#2070=CARTESIAN_POINT ( 'NONE',  ( 8.012675919994043991E-27, 44.00000000000019895, 2.908154216024726138E-28 ) ) ;
#2073=DIRECTION ( 'NONE',  ( 1.735493991486223169E-29, 0.000000000000000000, -1.000000000000000000 ) ) ;
#2074=ORIENTED_EDGE ( 'NONE', *, *, #586, .F. ) ;
#2078=CARTESIAN_POINT ( 'NONE',  ( -8.216777476527274970, 49.00000000000032685, -23.61111111111111427 ) ) ;
#2096=DIRECTION ( 'NONE',  ( -1.820952055660014662E-28, -1.000000000000000000, -7.038118388768679669E-30 ) ) ;
#2109=CARTESIAN_POINT ( 'NONE',  ( 8.677469957431129860E-27, 46.00000000000018474, -26.00000000000012790 ) ) ;
#2113=AXIS2_PLACEMENT_3D ( 'NONE', #4462, #8851, #2073 ) ;
#2116=EDGE_CURVE ( 'NONE', #9587, #6156, #2701, .T. ) ;
#2117=VERTEX_POINT ( 'NONE', #4352 ) ;
#2119=ORIENTED_EDGE ( 'NONE', *, *, #1000, .T. ) ;
#2126=VECTOR ( 'NONE', #3661, 1000.000000000000000 ) ;
#2148=PLANE ( 'NONE',  #7284 ) ;
#2167=PLANE ( 'NONE',  #3723 ) ;
#2174=( NAMED_UNIT ( * ) SI_UNIT ( $, .STERADIAN. ) SOLID_ANGLE_UNIT ( ) );
#2177=CIRCLE ( 'NONE', #7722, 26.00000000000003197 ) ;
#2178=DIRECTION ( 'NONE',  ( 0.9860132971832693549, 1.788557213313974126E-28, -0.1666666666666657970 ) ) ;
#2179=ADVANCED_FACE ( 'NONE', ( #1966 ), #8792, .F. ) ;
#2183=LINE ( 'NONE', #4392, #6528 ) ;
#2190=DIRECTION ( 'NONE',  ( 1.735493991486225411E-29, 0.000000000000000000, -1.000000000000000000 ) ) ;
#2192=VERTEX_POINT ( 'NONE', #5382 ) ;
#2194=LINE ( 'NONE', #5232, #1991 ) ;
#2198=DIRECTION ( 'NONE',  ( -0.3286710990610922090, -6.289316826390952918E-29, -0.9444444444444435316 ) ) ;
#2200=ORIENTED_EDGE ( 'NONE', *, *, #9573, .T. ) ;
#2205=DIRECTION ( 'NONE',  ( -1.820952055660014662E-28, -1.000000000000000000, -7.038118388768679669E-30 ) ) ;
#2218=ORIENTED_EDGE ( 'NONE', *, *, #4260, .T. ) ;
#2224=CARTESIAN_POINT ( 'NONE',  ( -8.216777476527274970, 78.08723716182652197, -23.61111111111111427 ) ) ;
#2233=CARTESIAN_POINT ( 'NONE',  ( 1.555535097482682654E-26, 78.08723716182652197, -25.00000000000000000 ) ) ;
#2238=VECTOR ( 'NONE', #3063, 1000.000000000000341 ) ;
#2242=ADVANCED_FACE ( 'NONE', ( #8190 ), #738, .F. ) ;
#2248=EDGE_CURVE ( 'NONE', #1081, #9622, #689, .T. ) ;
#2249=EDGE_CURVE ( 'NONE', #8507, #3257, #2892, .T. ) ;
#2263=CARTESIAN_POINT ( 'NONE',  ( 1.084683744678891232E-26, 56.00000000000030553, -26.00000000000003197 ) ) ;
#2264=ORIENTED_EDGE ( 'NONE', *, *, #8365, .F. ) ;
#2266=AXIS2_PLACEMENT_3D ( 'NONE', #3694, #2947, #2190 ) ;
#2267=VERTEX_POINT ( 'NONE', #6107 ) ;
#2277=UNCERTAINTY_MEASURE_WITH_UNIT (LENGTH_MEASURE( 1.000000000000000082E-05 ), #147, 'distance_accuracy_value', 'NONE');
#2302=DIRECTION ( 'NONE',  ( -1.735493991486225972E-29, 6.508102468073347395E-30, 1.000000000000000000 ) ) ;
#2313=DIRECTION ( 'NONE',  ( 1.735493991486225972E-29, -6.508102468073347395E-30, -1.000000000000000000 ) ) ;
#2316=CARTESIAN_POINT ( 'NONE',  ( 0.000000000000000000, 0.000000000000000000, 0.000000000000000000 ) ) ;
#2319=DIRECTION ( 'NONE',  ( -0.3286710990610922090, -6.289316826390952918E-29, -0.9444444444444435316 ) ) ;
#2329=EDGE_CURVE ( 'NONE', #1005, #5592, #4652, .T. ) ;
#2331=ORIENTED_EDGE ( 'NONE', *, *, #7093, .F. ) ;
#2335=ORIENTED_EDGE ( 'NONE', *, *, #1978, .F. ) ;
#2342=DIRECTION ( 'NONE',  ( -0.9860132971832694659, -1.788557213313974350E-28, 0.1666666666666658247 ) ) ;
#2345=CARTESIAN_POINT ( 'NONE',  ( -8.216777476527274970, 48.50000000000033396, -23.61111111111111427 ) ) ;
#2346=VECTOR ( 'NONE', #5667, 1000.000000000000000 ) ;
#2356=VECTOR ( 'NONE', #2178, 1000.000000000000341 ) ;
#2361=VECTOR ( 'NONE', #5255, 1000.000000000000000 ) ;
#2373=EDGE_CURVE ( 'NONE', #7030, #1931, #1675, .T. ) ;
#2385=ORIENTED_EDGE ( 'NONE', *, *, #3424, .T. ) ;
#2386=CARTESIAN_POINT ( 'NONE',  ( -8.545448575588387996, 47.00000000000034106, -24.55555555555564240 ) ) ;
#2387=LINE ( 'NONE', #1654, #6606 ) ;
#2396=VERTEX_POINT ( 'NONE', #1860 ) ;
#2399=DIRECTION ( 'NONE',  ( 1.735493991486225972E-29, -6.508102468073347395E-30, -1.000000000000000000 ) ) ;
#2401=DIRECTION ( 'NONE',  ( 0.3286710990610922090, 6.289316826390952918E-29, 0.9444444444444435316 ) ) ;
#2404=CIRCLE ( 'NONE', #7938, 26.00000000000015987 ) ;
#2415=FACE_OUTER_BOUND ( 'NONE', #2610, .T. ) ;
#2416=CARTESIAN_POINT ( 'NONE',  ( 1.040310318760209318E-26, 47.50000000000033396, -25.00000000000000000 ) ) ;
#2418=ADVANCED_FACE ( 'NONE', ( #7039 ), #4838, .T. ) ;
#2421=VERTEX_POINT ( 'NONE', #3290 ) ;
#2425=ORIENTED_EDGE ( 'NONE', *, *, #6649, .F. ) ;
#2434=AXIS2_PLACEMENT_3D ( 'NONE', #1777, #1044, #5681 ) ;
#2439=ADVANCED_FACE ( 'NONE', ( #2450 ), #5484, .F. ) ;
#2441=EDGE_CURVE ( 'NONE', #6423, #9611, #8638, .T. ) ;
#2442=DIRECTION ( 'NONE',  ( 1.735493991486225972E-29, -6.508102468073347395E-30, -1.000000000000000000 ) ) ;
#2443=VERTEX_POINT ( 'NONE', #6155 ) ;
#2444=EDGE_CURVE ( 'NONE', #7011, #3069, #1027, .T. ) ;
#2448=AXIS2_PLACEMENT_3D ( 'NONE', #1107, #7122, #4077 ) ;
#2449=VECTOR ( 'NONE', #6864, 1000.000000000000227 ) ;
#2450=FACE_OUTER_BOUND ( 'NONE', #3947, .T. ) ;
#2451=EDGE_CURVE ( 'NONE', #5638, #478, #6208, .T. ) ;
#2456=DIRECTION ( 'NONE',  ( -1.820952055660014662E-28, -1.000000000000000000, -7.038118388768679669E-30 ) ) ;
#2470=ORIENTED_EDGE ( 'NONE', *, *, #7272, .F. ) ;
#2471=DIRECTION ( 'NONE',  ( 1.735493991486225972E-29, -6.508102468073347395E-30, -1.000000000000000000 ) ) ;
#2472=ORIENTED_EDGE ( 'NONE', *, *, #2805, .T. ) ;
#2476=CARTESIAN_POINT ( 'NONE',  ( 1.030449557444946671E-26, 53.00000000000031974, -26.00000000000006395 ) ) ;
#2485=CARTESIAN_POINT ( 'NONE',  ( 1.555535097482682654E-26, 78.08723716182652197, -25.00000000000000000 ) ) ;
#2487=EDGE_CURVE ( 'NONE', #4270, #9611, #6368, .T. ) ;
#2497=ADVANCED_FACE ( 'NONE', ( #4146 ), #2049, .F. ) ;
#2504=EDGE_LOOP ( 'NONE', ( #8119, #8136, #5007, #6177 ) ) ;
#2505=CARTESIAN_POINT ( 'NONE',  ( -8.545448575588384443, 48.50000000000033396, -24.55555555555566727 ) ) ;
#2512=ORIENTED_EDGE ( 'NONE', *, *, #930, .F. ) ;
#2514=ORIENTED_EDGE ( 'NONE', *, *, #2451, .F. ) ;
#2520=PLANE ( 'NONE',  #2448 ) ;
#2526=VECTOR ( 'NONE', #1753, 1000.000000000000000 ) ;
#2528=DIRECTION ( 'NONE',  ( -1.820952055660014662E-28, -1.000000000000000000, 6.508102468073347395E-30 ) ) ;
#2533=DIRECTION ( 'NONE',  ( 1.735493991486228775E-29, 0.000000000000000000, -1.000000000000000000 ) ) ;
#2535=VECTOR ( 'NONE', #5235, 1000.000000000000341 ) ;
#2537=VERTEX_POINT ( 'NONE', #2839 ) ;
#2539=DIRECTION ( 'NONE',  ( -0.9860132971832693549, -1.788557213313974126E-28, 0.1666666666666657970 ) ) ;
#2542=CARTESIAN_POINT ( 'NONE',  ( -8.545448575588386220, -1.757603667247791439E-27, -24.55555555555562108 ) ) ;
#2545=VECTOR ( 'NONE', #6775, 1000.000000000000000 ) ;
#2559=ORIENTED_EDGE ( 'NONE', *, *, #3022, .F. ) ;
#2563=CARTESIAN_POINT ( 'NONE',  ( 5.423418723394456162E-28, -2.066522830327504070E-28, -26.00000000000012790 ) ) ;
#2564=CARTESIAN_POINT ( 'NONE',  ( 1.099474886651785204E-26, 54.50000000000031264, -37.00000000000000711 ) ) ;
#2593=PRODUCT ( 'Hardened Alloy Threading Chaser Dies', 'Hardened Alloy Threading Chaser Dies', '', ( #2958 ) ) ;
#2603=CARTESIAN_POINT ( 'NONE',  ( 9.318419442923201951E-27, 44.00000000000019895, -25.00000000000000000 ) ) ;
#2610=EDGE_LOOP ( 'NONE', ( #9034, #3632, #8949, #660 ) ) ;
#2614=CARTESIAN_POINT ( 'NONE',  ( -8.545448575588386220, 46.00000000000018474, -24.55555555555567793 ) ) ;
#2615=CARTESIAN_POINT ( 'NONE',  ( -8.216777476527294510, 51.50000000000032685, -23.61111111111107519 ) ) ;
#2621=ORIENTED_EDGE ( 'NONE', *, *, #3022, .T. ) ;
#2623=EDGE_CURVE ( 'NONE', #7113, #6031, #2183, .T. ) ;
#2625=CARTESIAN_POINT ( 'NONE',  ( -8.545448575588366680, 58.00000000000029132, -24.55555555555552161 ) ) ;
#2627=ORIENTED_EDGE ( 'NONE', *, *, #7508, .F. ) ;
#2634=DIRECTION ( 'NONE',  ( 1.820952055660014662E-28, 1.000000000000000000, -6.508102468073347395E-30 ) ) ;
#2635=DIRECTION ( 'NONE',  ( -0.9860132971832693549, -1.788557213313974126E-28, 0.1666666666666657970 ) ) ;
#2637=PLANE ( 'NONE',  #7435 ) ;
#2646=EDGE_CURVE ( 'NONE', #3069, #6892, #8333, .T. ) ;
#2650=ORIENTED_EDGE ( 'NONE', *, *, #8232, .T. ) ;
#2657=AXIS2_PLACEMENT_3D ( 'NONE', #8324, #5893, #9653 ) ;
#2674=EDGE_CURVE ( 'NONE', #6976, #2267, #1565, .T. ) ;
#2682=CARTESIAN_POINT ( 'NONE',  ( 9.762153702110021092E-27, 53.00000000000031974, -24.09806918451527835 ) ) ;
#2684=AXIS2_PLACEMENT_3D ( 'NONE', #6033, #1605, #7683 ) ;
#2685=EDGE_CURVE ( 'NONE', #9391, #7720, #7395, .T. ) ;
#2686=DIRECTION ( 'NONE',  ( -0.9860132971832694659, -1.788557213313974350E-28, 0.1666666666666658247 ) ) ;
#2687=EDGE_CURVE ( 'NONE', #4799, #49, #104, .T. ) ;
#2693=ORIENTED_EDGE ( 'NONE', *, *, #3729, .F. ) ;
#2700=ORIENTED_EDGE ( 'NONE', *, *, #3775, .T. ) ;
#2701=LINE ( 'NONE', #3599, #5449 ) ;
#2710=VECTOR ( 'NONE', #5961, 1000.000000000000341 ) ;
#2714=VERTEX_POINT ( 'NONE', #9077 ) ;
#2716=VERTEX_POINT ( 'NONE', #7442 ) ;
#2731=VERTEX_POINT ( 'NONE', #7220 ) ;
#2734=CARTESIAN_POINT ( 'NONE',  ( 1.555535097482682654E-26, 78.08723716182652197, -25.00000000000000000 ) ) ;
#2735=DIRECTION ( 'NONE',  ( -1.820952055660014662E-28, -1.000000000000000000, -7.038118388768679669E-30 ) ) ;
#2747=ORIENTED_EDGE ( 'NONE', *, *, #4451, .F. ) ;
#2764=VECTOR ( 'NONE', #6634, 1000.000000000000000 ) ;
#2765=AXIS2_PLACEMENT_3D ( 'NONE', #6760, #3208, #1693 ) ;
#2769=ORIENTED_EDGE ( 'NONE', *, *, #7915, .T. ) ;
#2776=ORIENTED_EDGE ( 'NONE', *, *, #8975, .T. ) ;
#2780=ORIENTED_EDGE ( 'NONE', *, *, #6900, .F. ) ;
#2794=FACE_OUTER_BOUND ( 'NONE', #6929, .T. ) ;
#2797=ADVANCED_FACE ( 'NONE', ( #1843 ), #4859, .F. ) ;
#2805=EDGE_CURVE ( 'NONE', #4022, #2912, #7922, .T. ) ;
#2821=CARTESIAN_POINT ( 'NONE',  ( -8.216777476527294510, 57.50000000000029843, -23.61111111111111427 ) ) ;
#2825=LINE ( 'NONE', #8120, #6231 ) ;
#2827=CARTESIAN_POINT ( 'NONE',  ( 5.423418723394456162E-28, -2.066522830327504070E-28, -26.00000000000017408 ) ) ;
#2828=EDGE_CURVE ( 'NONE', #4569, #2443, #4124, .T. ) ;
#2830=DIRECTION ( 'NONE',  ( 0.000000000000000000, 0.000000000000000000, 1.000000000000000000 ) ) ;
#2833=CARTESIAN_POINT ( 'NONE',  ( 1.094544505994153880E-26, 57.50000000000029843, -24.09806918451523217 ) ) ;
#2834=VECTOR ( 'NONE', #3680, 1000.000000000000000 ) ;
#2839=CARTESIAN_POINT ( 'NONE',  ( -8.216777476527294510, 50.50000000000031974, -23.61111111111111427 ) ) ;
#2846=AXIS2_PLACEMENT_3D ( 'NONE', #5612, #1117, #1853 ) ;
#2847=PRODUCT_DEFINITION_FORMATION_WITH_SPECIFIED_SOURCE ( 'ANY', '', #2593, .NOT_KNOWN. ) ;
#2848=VERTEX_POINT ( 'NONE', #2625 ) ;
#2857=VERTEX_POINT ( 'NONE', #7825 ) ;
#2864=CARTESIAN_POINT ( 'NONE',  ( 1.084683744678891232E-26, 58.00000000000029132, -26.00000000000000355 ) ) ;
#2873=VERTEX_POINT ( 'NONE', #2864 ) ;
#2874=DIRECTION ( 'NONE',  ( -1.820952055660014662E-28, -1.000000000000000000, -7.038118388768679669E-30 ) ) ;
#2888=DIRECTION ( 'NONE',  ( 1.820952055660014662E-28, 1.000000000000000000, 7.038118388768679669E-30 ) ) ;
#2892=LINE ( 'NONE', #110, #1174 ) ;
#2893=ORIENTED_EDGE ( 'NONE', *, *, #1774, .F. ) ;
#2897=AXIS2_PLACEMENT_3D ( 'NONE', #3347, #1231, #496 ) ;
#2899=CARTESIAN_POINT ( 'NONE',  ( 9.860761315262647568E-27, 51.50000000000032685, -26.00000000000008171 ) ) ;
#2906=VECTOR ( 'NONE', #7189, 1000.000000000000000 ) ;
#2912=VERTEX_POINT ( 'NONE', #5879 ) ;
#2915=CIRCLE ( 'NONE', #9393, 26.00000000000012790 ) ;
#2919=CARTESIAN_POINT ( 'NONE',  ( 1.040310318760209318E-26, 51.50000000000032685, -25.00000000000000000 ) ) ;
#2925=EDGE_CURVE ( 'NONE', #77, #3257, #4312, .T. ) ;
#2926=EDGE_CURVE ( 'NONE', #9428, #3135, #1497, .T. ) ;
#2938=ORIENTED_EDGE ( 'NONE', *, *, #7225, .F. ) ;
#2942=CARTESIAN_POINT ( 'NONE',  ( 1.148778693228098442E-26, 59.00000000000029843, -26.00000000000000355 ) ) ;
#2947=DIRECTION ( 'NONE',  ( -1.820952055660014662E-28, -1.000000000000000000, -7.038118388768679669E-30 ) ) ;
#2949=VERTEX_POINT ( 'NONE', #4409 ) ;
#2956=EDGE_CURVE ( 'NONE', #9742, #9391, #8804, .T. ) ;
#2958=PRODUCT_CONTEXT ( 'NONE', #4296, 'mechanical' ) ;
#2974=ADVANCED_FACE ( 'NONE', ( #5446 ), #3760, .F. ) ;
#2976=CARTESIAN_POINT ( 'NONE',  ( 0.000000000000000000, 0.000000000000000000, 0.000000000000000000 ) ) ;
#2986=CARTESIAN_POINT ( 'NONE',  ( -8.216777476527294510, 42.50000000000020606, -23.61111111111107519 ) ) ;
#2993=CARTESIAN_POINT ( 'NONE',  ( 1.555535097482682654E-26, 78.08723716182652197, -25.00000000000000000 ) ) ;
#2995=LINE ( 'NONE', #8239, #8390 ) ;
#3005=ORIENTED_EDGE ( 'NONE', *, *, #4933, .T. ) ;
#3006=DIRECTION ( 'NONE',  ( 1.735493991486226532E-29, 0.000000000000000000, -1.000000000000000000 ) ) ;
#3010=DIRECTION ( 'NONE',  ( 1.735493991486225972E-29, -6.508102468073347395E-30, -1.000000000000000000 ) ) ;
#3015=VECTOR ( 'NONE', #1290, 1000.000000000000341 ) ;
#3021=CYLINDRICAL_SURFACE ( 'NONE', #7482, 26.00000000000003197 ) ;
#3022=EDGE_CURVE ( 'NONE', #2714, #1495, #7331, .T. ) ;
#3025=CARTESIAN_POINT ( 'NONE',  ( -8.545448575588366680, -1.757025888264475269E-27, -24.55555555555556424 ) ) ;
#3031=LINE ( 'NONE', #2986, #5852 ) ;
#3034=CARTESIAN_POINT ( 'NONE',  ( 1.030449557444946671E-26, 48.50000000000033396, -25.00000000000000000 ) ) ;
#3035=CARTESIAN_POINT ( 'NONE',  ( 0.000000000000000000, 0.000000000000000000, 0.000000000000000000 ) ) ;
#3036=EDGE_LOOP ( 'NONE', ( #1378, #1929, #3940, #8036 ) ) ;
#3038=EDGE_CURVE ( 'NONE', #5882, #9092, #906, .T. ) ;
#3042=ORIENTED_EDGE ( 'NONE', *, *, #7891, .T. ) ;
#3045=VERTEX_POINT ( 'NONE', #1482 ) ;
#3046=LINE ( 'NONE', #5338, #3501 ) ;
#3047=VECTOR ( 'NONE', #2539, 1000.000000000000341 ) ;
#3054=DIRECTION ( 'NONE',  ( 1.735493991486226532E-29, 0.000000000000000000, -1.000000000000000000 ) ) ;
#3058=CARTESIAN_POINT ( 'NONE',  ( 1.030449557444946671E-26, 48.50000000000033396, -25.00000000000000000 ) ) ;
#3062=PLANE ( 'NONE',  #2765 ) ;
#3063=DIRECTION ( 'NONE',  ( -0.9860132971832693549, -1.788557213313974126E-28, 0.1666666666666657970 ) ) ;
#3065=AXIS2_PLACEMENT_3D ( 'NONE', #4972, #9318, #2533 ) ;
#3069=VERTEX_POINT ( 'NONE', #7615 ) ;
#3070=VECTOR ( 'NONE', #5407, 1000.000000000000000 ) ;
#3079=ORIENTED_EDGE ( 'NONE', *, *, #3207, .F. ) ;
#3082=VERTEX_POINT ( 'NONE', #2263 ) ;
#3087=CARTESIAN_POINT ( 'NONE',  ( 9.860761315262647568E-27, 47.50000000000033396, -24.09806918451532809 ) ) ;
#3091=VECTOR ( 'NONE', #9294, 1000.000000000000341 ) ;
#3097=EDGE_LOOP ( 'NONE', ( #8573, #8616, #5009, #2627 ) ) ;
#3101=DIRECTION ( 'NONE',  ( 0.3286710990610922090, 6.289316826390952918E-29, 0.9444444444444435316 ) ) ;
#3107=DIRECTION ( 'NONE',  ( -0.3286710990610922090, -6.289316826390952918E-29, -0.9444444444444435316 ) ) ;
#3125=ORIENTED_EDGE ( 'NONE', *, *, #7989, .T. ) ;
#3126=LINE ( 'NONE', #773, #1583 ) ;
#3132=DIRECTION ( 'NONE',  ( -1.820952055660014662E-28, -1.000000000000000000, -7.038118388768679669E-30 ) ) ;
#3135=VERTEX_POINT ( 'NONE', #7155 ) ;
#3136=DIRECTION ( 'NONE',  ( -1.820952055660014662E-28, -1.000000000000000000, -7.038118388768679669E-30 ) ) ;
#3160=AXIS2_PLACEMENT_3D ( 'NONE', #3234, #3790, #6789 ) ;
#3169=EDGE_CURVE ( 'NONE', #5882, #6521, #3411, .T. ) ;
#3181=DIRECTION ( 'NONE',  ( -1.820952055660014662E-28, -1.000000000000000000, -7.038118388768679669E-30 ) ) ;
#3182=VECTOR ( 'NONE', #9042, 1000.000000000000341 ) ;
#3184=FACE_OUTER_BOUND ( 'NONE', #3036, .T. ) ;
#3187=EDGE_LOOP ( 'NONE', ( #1746, #9733, #5763, #2026 ) ) ;
#3198=LINE ( 'NONE', #7860, #9345 ) ;
#3199=LINE ( 'NONE', #158, #7823 ) ;
#3207=EDGE_CURVE ( 'NONE', #8853, #9742, #4347, .T. ) ;
#3208=DIRECTION ( 'NONE',  ( -1.820952055660014662E-28, -1.000000000000000000, 6.508102468073347395E-30 ) ) ;
#3225=VERTEX_POINT ( 'NONE', #994 ) ;
#3228=VECTOR ( 'NONE', #3991, 1000.000000000000000 ) ;
#3230=LINE ( 'NONE', #6285, #6793 ) ;
#3234=CARTESIAN_POINT ( 'NONE',  ( 9.101986939180200354E-27, 50.00000000000032685, 2.962080254467568742E-28 ) ) ;
#3237=CARTESIAN_POINT ( 'NONE',  ( 1.257247067695987565E-26, 60.00000000000029843, -37.00000000000000711 ) ) ;
#3243=VECTOR ( 'NONE', #5299, 1000.000000000000341 ) ;
#3245=CARTESIAN_POINT ( 'NONE',  ( 1.075405720943667276E-26, 59.00000000000029843, 3.085339770908351837E-28 ) ) ;
#3249=VERTEX_POINT ( 'NONE', #5583 ) ;
#3255=EDGE_LOOP ( 'NONE', ( #6378, #8612, #9181, #9132 ) ) ;
#3257=VERTEX_POINT ( 'NONE', #214 ) ;
#3265=DIRECTION ( 'NONE',  ( 0.9860132971832693549, 1.788557213313974126E-28, -0.1666666666666657970 ) ) ;
#3273=FACE_OUTER_BOUND ( 'NONE', #6199, .T. ) ;
#3284=EDGE_CURVE ( 'NONE', #5419, #4022, #4356, .T. ) ;
#3287=EDGE_CURVE ( 'NONE', #2731, #8853, #4300, .T. ) ;
#3290=CARTESIAN_POINT ( 'NONE',  ( -8.216777476527294510, 51.50000000000032685, -23.61111111111107519 ) ) ;
#3295=ORIENTED_EDGE ( 'NONE', *, *, #9390, .F. ) ;
#3300=AXIS2_PLACEMENT_3D ( 'NONE', #1996, #7984, #9606 ) ;
#3302=AXIS2_PLACEMENT_3D ( 'NONE', #746, #1336, #7414 ) ;
#3316=ORIENTED_EDGE ( 'NONE', *, *, #7237, .T. ) ;
#3318=ORIENTED_EDGE ( 'NONE', *, *, #1549, .F. ) ;
#3321=ORIENTED_EDGE ( 'NONE', *, *, #2674, .F. ) ;
#3324=DIRECTION ( 'NONE',  ( 1.820952055660014662E-28, 1.000000000000000000, -6.508102468073347395E-30 ) ) ;
#3325=LINE ( 'NONE', #8667, #4158 ) ;
#3326=ORIENTED_EDGE ( 'NONE', *, *, #553, .F. ) ;
#3327=LINE ( 'NONE', #7127, #7412 ) ;
#3331=ORIENTED_EDGE ( 'NONE', *, *, #255, .T. ) ;
#3335=CARTESIAN_POINT ( 'NONE',  ( 1.555535097482682654E-26, 78.08723716182652197, -25.00000000000000000 ) ) ;
#3336=DIRECTION ( 'NONE',  ( 1.820952055660014662E-28, 1.000000000000000000, -6.508102468073347395E-30 ) ) ;
#3339=AXIS2_PLACEMENT_3D ( 'NONE', #6651, #8945, #647 ) ;
#3342=CARTESIAN_POINT ( 'NONE',  ( 8.233735698244310719E-27, 44.00000000000019895, -24.09806918451537072 ) ) ;
#3347=CARTESIAN_POINT ( 'NONE',  ( 1.555535097482682654E-26, 78.08723716182652197, -25.00000000000000000 ) ) ;
#3351=EDGE_CURVE ( 'NONE', #2873, #8065, #5782, .T. ) ;
#3354=DIRECTION ( 'NONE',  ( -1.820952055660014662E-28, -1.000000000000000000, -7.038118388768679669E-30 ) ) ;
#3355=VECTOR ( 'NONE', #7322, 1000.000000000000000 ) ;
#3357=VECTOR ( 'NONE', #4197, 1000.000000000000000 ) ;
#3361=ORIENTED_EDGE ( 'NONE', *, *, #7270, .F. ) ;
#3364=DIRECTION ( 'NONE',  ( -0.9860132971832693549, -1.788557213313974126E-28, 0.1666666666666657970 ) ) ;
#3370=EDGE_LOOP ( 'NONE', ( #7116, #8619, #4183, #2747 ) ) ;
#3386=FACE_OUTER_BOUND ( 'NONE', #4037, .T. ) ;
#3396=CARTESIAN_POINT ( 'NONE',  ( -8.545448575588398654, 43.00000000000019895, -24.55555555555570990 ) ) ;
#3398=ORIENTED_EDGE ( 'NONE', *, *, #8007, .T. ) ;
#3399=VECTOR ( 'NONE', #4586, 1000.000000000000000 ) ;
#3411=LINE ( 'NONE', #3960, #7805 ) ;
#3415=VERTEX_POINT ( 'NONE', #9672 ) ;
#3419=FACE_OUTER_BOUND ( 'NONE', #3969, .T. ) ;
#3424=EDGE_CURVE ( 'NONE', #7994, #517, #5821, .T. ) ;
#3431=DIRECTION ( 'NONE',  ( -1.735493991486225972E-29, 6.508102468073347395E-30, 1.000000000000000000 ) ) ;
#3435=ORIENTED_EDGE ( 'NONE', *, *, #464, .T. ) ;
#3443=LINE ( 'NONE', #544, #6234 ) ;
#3446=CARTESIAN_POINT ( 'NONE',  ( 1.040310318760209318E-26, 56.50000000000029843, -24.09806918451523217 ) ) ;
#3452=ORIENTED_EDGE ( 'NONE', *, *, #8538, .T. ) ;
#3459=LINE ( 'NONE', #2615, #5457 ) ;
#3461=EDGE_CURVE ( 'NONE', #4048, #5730, #1525, .T. ) ;
#3476=EDGE_CURVE ( 'NONE', #5730, #7381, #2995, .T. ) ;
#3480=ORIENTED_EDGE ( 'NONE', *, *, #107, .T. ) ;
#3490=CARTESIAN_POINT ( 'NONE',  ( 9.811457508686334330E-27, 52.00000000000031974, -24.09806918451527835 ) ) ;
#3493=CARTESIAN_POINT ( 'NONE',  ( 9.269115636346888714E-27, 44.00000000000019895, -26.00000000000015987 ) ) ;
#3499=CARTESIAN_POINT ( 'NONE',  ( -8.216777476527294510, 56.00000000000030553, -23.61111111111111427 ) ) ;
#3501=VECTOR ( 'NONE', #2456, 1000.000000000000000 ) ;
#3503=CARTESIAN_POINT ( 'NONE',  ( 1.099474886651785204E-26, 54.50000000000031264, -25.00000000000000000 ) ) ;
#3527=DIRECTION ( 'NONE',  ( -1.820952055660014662E-28, -1.000000000000000000, -7.038118388768679669E-30 ) ) ;
#3536=ORIENTED_EDGE ( 'NONE', *, *, #8678, .F. ) ;
#3541=ORIENTED_EDGE ( 'NONE', *, *, #890, .F. ) ;
#3542=DIRECTION ( 'NONE',  ( -1.820952055660014662E-28, -1.000000000000000000, 6.508102468073347395E-30 ) ) ;
#3543=DIRECTION ( 'NONE',  ( -1.735493991486225972E-29, 6.508102468073347395E-30, 1.000000000000000000 ) ) ;
#3547=LINE ( 'NONE', #2224, #47 ) ;
#3557=CARTESIAN_POINT ( 'NONE',  ( -8.545448575588386220, 53.00000000000031974, -24.55555555555562108 ) ) ;
#3562=EDGE_CURVE ( 'NONE', #1238, #6156, #6698, .T. ) ;
#3577=ORIENTED_EDGE ( 'NONE', *, *, #8678, .T. ) ;
#3595=CARTESIAN_POINT ( 'NONE',  ( -8.545448575588393325, -1.754907365325649309E-27, -24.55555555555563529 ) ) ;
#3599=CARTESIAN_POINT ( 'NONE',  ( -8.216777476527274970, 78.08723716182652197, -23.61111111111111427 ) ) ;
#3606=ORIENTED_EDGE ( 'NONE', *, *, #226, .T. ) ;
#3613=ORIENTED_EDGE ( 'NONE', *, *, #5889, .F. ) ;
#3624=VERTEX_POINT ( 'NONE', #5432 ) ;
#3626=DIRECTION ( 'NONE',  ( -0.1666666666666658525, -3.897465909857536228E-29, -0.9860132971832695770 ) ) ;
#3627=CARTESIAN_POINT ( 'NONE',  ( 1.084683744678891232E-26, 53.50000000000031264, -25.00000000000000000 ) ) ;
#3632=ORIENTED_EDGE ( 'NONE', *, *, #5051, .F. ) ;
#3634=DIRECTION ( 'NONE',  ( 1.735493991486225972E-29, -6.508102468073347395E-30, -1.000000000000000000 ) ) ;
#3641=DIRECTION ( 'NONE',  ( 1.820952055660014662E-28, 1.000000000000000000, 7.038118388768679669E-30 ) ) ;
#3661=DIRECTION ( 'NONE',  ( -1.820952055660014662E-28, -1.000000000000000000, -7.038118388768679669E-30 ) ) ;
#3669=VECTOR ( 'NONE', #9069, 1000.000000000000000 ) ;
#3671=ORIENTED_EDGE ( 'NONE', *, *, #3284, .T. ) ;
#3672=CYLINDRICAL_SURFACE ( 'NONE', #652, 26.00000000000015987 ) ;
#3673=ORIENTED_EDGE ( 'NONE', *, *, #3476, .F. ) ;
#3676=( LENGTH_UNIT ( ) NAMED_UNIT ( * ) SI_UNIT ( .MILLI., .METRE. ) );
#3677=CARTESIAN_POINT ( 'NONE',  ( 8.283655523829511658E-27, 45.50000000000019185, 2.877339336914530364E-28 ) ) ;
#3678=DIRECTION ( 'NONE',  ( -0.9860132971832693549, -1.788557213313974126E-28, 0.1666666666666657970 ) ) ;
#3680=DIRECTION ( 'NONE',  ( 1.735493991486225972E-29, -6.508102468073347395E-30, -1.000000000000000000 ) ) ;
#3682=VERTEX_POINT ( 'NONE', #3396 ) ;
#3684=CARTESIAN_POINT ( 'NONE',  ( -12.16083066526041989, 40.00000000000014921, -34.94444444444444287 ) ) ;
#3688=FACE_OUTER_BOUND ( 'NONE', #7634, .T. ) ;
#3694=CARTESIAN_POINT ( 'NONE',  ( 9.754302352884585496E-27, 53.50000000000031264, 3.158525108795066799E-28 ) ) ;
#3701=CARTESIAN_POINT ( 'NONE',  ( 1.040310318760209318E-26, 51.50000000000032685, -25.00000000000000000 ) ) ;
#3702=CARTESIAN_POINT ( 'NONE',  ( -8.545448575588372009, 57.50000000000029843, -24.55555555555557845 ) ) ;
#3715=ORIENTED_EDGE ( 'NONE', *, *, #9204, .F. ) ;
#3716=LINE ( 'NONE', #3058, #3243 ) ;
#3723=AXIS2_PLACEMENT_3D ( 'NONE', #615, #4272, #7377 ) ;
#3724=LINE ( 'NONE', #2821, #7296 ) ;
#3727=ORIENTED_EDGE ( 'NONE', *, *, #1788, .T. ) ;
#3729=EDGE_CURVE ( 'NONE', #1008, #7461, #9476, .T. ) ;
#3731=DIRECTION ( 'NONE',  ( -1.820952055660014662E-28, -1.000000000000000000, -7.038118388768679669E-30 ) ) ;
#3742=DIRECTION ( 'NONE',  ( 1.735493991486225972E-29, -6.508102468073347395E-30, -1.000000000000000000 ) ) ;
#3745=EDGE_CURVE ( 'NONE', #6660, #2267, #4394, .T. ) ;
#3748=ORIENTED_EDGE ( 'NONE', *, *, #6649, .T. ) ;
#3752=LINE ( 'NONE', #4499, #2710 ) ;
#3757=ORIENTED_EDGE ( 'NONE', *, *, #2444, .F. ) ;
#3759=LINE ( 'NONE', #3861, #631 ) ;
#3760=CYLINDRICAL_SURFACE ( 'NONE', #4503, 26.00000000000009592 ) ;
#3772=ORIENTED_EDGE ( 'NONE', *, *, #7514, .T. ) ;
#3773=DIRECTION ( 'NONE',  ( 1.735493991486225972E-29, -6.508102468073347395E-30, -1.000000000000000000 ) ) ;
#3775=EDGE_CURVE ( 'NONE', #3682, #3950, #2404, .T. ) ;
#3777=EDGE_CURVE ( 'NONE', #8006, #5592, #8141, .T. ) ;
#3778=ADVANCED_FACE ( 'NONE', ( #9615 ), #4344, .F. ) ;
#3784=ORIENTED_EDGE ( 'NONE', *, *, #7529, .T. ) ;
#3786=DIRECTION ( 'NONE',  ( 1.820952055660014662E-28, 1.000000000000000000, 7.038118388768679669E-30 ) ) ;
#3790=DIRECTION ( 'NONE',  ( -1.820952055660014662E-28, -1.000000000000000000, -7.038118388768679669E-30 ) ) ;
#3792=EDGE_LOOP ( 'NONE', ( #24, #1953, #3835, #2074 ) ) ;
#3795=VECTOR ( 'NONE', #8173, 1000.000000000000341 ) ;
#3796=CARTESIAN_POINT ( 'NONE',  ( 9.860761315262647568E-27, 51.50000000000032685, -24.09806918451529612 ) ) ;
#3809=CARTESIAN_POINT ( 'NONE',  ( 1.099474886651785204E-26, 54.50000000000031264, -25.00000000000000000 ) ) ;
#3810=CARTESIAN_POINT ( 'NONE',  ( 8.677469957431129860E-27, 43.00000000000019895, -25.00000000000000000 ) ) ;
#3814=ORIENTED_EDGE ( 'NONE', *, *, #7989, .F. ) ;
#3824=VERTEX_POINT ( 'NONE', #5769 ) ;
#3826=VECTOR ( 'NONE', #5722, 1000.000000000000000 ) ;
#3827=CYLINDRICAL_SURFACE ( 'NONE', #9397, 26.00000000000017408 ) ;
#3835=ORIENTED_EDGE ( 'NONE', *, *, #5056, .T. ) ;
#3843=CARTESIAN_POINT ( 'NONE',  ( 5.423418723394456162E-28, -2.066522830327504070E-28, -26.00000000000011369 ) ) ;
#3844=LINE ( 'NONE', #8883, #1102 ) ;
#3848=ADVANCED_FACE ( 'NONE', ( #7243 ), #495, .F. ) ;
#3854=VECTOR ( 'NONE', #1717, 1000.000000000000000 ) ;
#3855=DIRECTION ( 'NONE',  ( -1.735493991486225972E-29, 6.508102468073347395E-30, 1.000000000000000000 ) ) ;
#3858=ORIENTED_EDGE ( 'NONE', *, *, #821, .T. ) ;
#3861=CARTESIAN_POINT ( 'NONE',  ( -8.216777476527294510, 50.50000000000031974, -23.61111111111111427 ) ) ;
#3864=LINE ( 'NONE', #8407, #7988 ) ;
#3866=ORIENTED_EDGE ( 'NONE', *, *, #6900, .T. ) ;
#3870=EDGE_CURVE ( 'NONE', #4799, #5636, #6594, .T. ) ;
#3873=VERTEX_POINT ( 'NONE', #6552 ) ;
#3879=VECTOR ( 'NONE', #3265, 1000.000000000000341 ) ;
#3880=ORIENTED_EDGE ( 'NONE', *, *, #1672, .T. ) ;
#3882=FACE_OUTER_BOUND ( 'NONE', #8268, .T. ) ;
#3886=CIRCLE ( 'NONE', #5145, 26.00000000000011369 ) ;
#3889=CARTESIAN_POINT ( 'NONE',  ( -8.545448575588396878, 50.00000000000032685, -24.55555555555564951 ) ) ;
#3901=AXIS2_PLACEMENT_3D ( 'NONE', #9616, #1132, #393 ) ;
#3909=ADVANCED_FACE ( 'NONE', ( #5325 ), #2148, .F. ) ;
#3919=FACE_OUTER_BOUND ( 'NONE', #8691, .T. ) ;
#3924=ORIENTED_EDGE ( 'NONE', *, *, #4335, .F. ) ;
#3935=DIRECTION ( 'NONE',  ( -1.735493991486225972E-29, 6.508102468073347395E-30, 1.000000000000000000 ) ) ;
#3939=FACE_OUTER_BOUND ( 'NONE', #6860, .T. ) ;
#3940=ORIENTED_EDGE ( 'NONE', *, *, #1898, .T. ) ;
#3942=VECTOR ( 'NONE', #5043, 1000.000000000000000 ) ;
#3947=EDGE_LOOP ( 'NONE', ( #3536, #7222, #1850, #2693 ) ) ;
#3950=VERTEX_POINT ( 'NONE', #7444 ) ;
#3951=DIRECTION ( 'NONE',  ( -1.820952055660014662E-28, -1.000000000000000000, -7.038118388768679669E-30 ) ) ;
#3960=CARTESIAN_POINT ( 'NONE',  ( 1.636886378333599496E-26, 78.08723716182652197, -37.00000000000000711 ) ) ;
#3969=EDGE_LOOP ( 'NONE', ( #3673, #1043, #7126, #2264 ) ) ;
#3971=ORIENTED_EDGE ( 'NONE', *, *, #7518, .F. ) ;
#3991=DIRECTION ( 'NONE',  ( 1.735493991486225972E-29, -6.508102468073347395E-30, -1.000000000000000000 ) ) ;
#3998=VECTOR ( 'NONE', #4230, 1000.000000000000000 ) ;
#3999=ORIENTED_EDGE ( 'NONE', *, *, #7201, .T. ) ;
#4004=DIRECTION ( 'NONE',  ( 0.3286710990610922090, 6.289316826390952918E-29, 0.9444444444444435316 ) ) ;
#4020=CARTESIAN_POINT ( 'NONE',  ( -8.545448575588418194, -1.752788842386823350E-27, -24.55555555555570990 ) ) ;
#4022=VERTEX_POINT ( 'NONE', #4687 ) ;
#4034=DIRECTION ( 'NONE',  ( -1.820952055660014662E-28, -1.000000000000000000, -7.038118388768679669E-30 ) ) ;
#4037=EDGE_LOOP ( 'NONE', ( #7301, #8104, #2200, #5784 ) ) ;
#4046=VECTOR ( 'NONE', #659, 1000.000000000000000 ) ;
#4048=VERTEX_POINT ( 'NONE', #7786 ) ;
#4067=DIRECTION ( 'NONE',  ( 1.820952055660014662E-28, 1.000000000000000000, -6.508102468073347395E-30 ) ) ;
#4068=EDGE_CURVE ( 'NONE', #517, #6620, #146, .T. ) ;
#4070=ORIENTED_EDGE ( 'NONE', *, *, #3424, .F. ) ;
#4075=EDGE_LOOP ( 'NONE', ( #1164, #5691, #9036, #8341 ) ) ;
#4077=DIRECTION ( 'NONE',  ( -0.9860132971832694659, -1.788557213313974350E-28, 0.1666666666666658247 ) ) ;
#4083=CARTESIAN_POINT ( 'NONE',  ( 1.035379938102577995E-26, 54.50000000000031264, -24.09806918451526414 ) ) ;
#4084=CARTESIAN_POINT ( 'NONE',  ( 5.423418723394456162E-28, -2.066522830327504070E-28, -26.00000000000008171 ) ) ;
#4087=DIRECTION ( 'NONE',  ( -0.1666666666666658525, -3.897465909857536228E-29, -0.9860132971832695770 ) ) ;
#4093=ORIENTED_EDGE ( 'NONE', *, *, #7940, .T. ) ;
#4119=CIRCLE ( 'NONE', #9628, 26.00000000000014566 ) ;
#4124=LINE ( 'NONE', #1154, #8607 ) ;
#4132=DIRECTION ( 'NONE',  ( -1.735493991486225972E-29, 6.508102468073347395E-30, 1.000000000000000000 ) ) ;
#4133=CARTESIAN_POINT ( 'NONE',  ( -8.216777476527294510, 41.50000000000020606, -23.61111111111111427 ) ) ;
#4135=CARTESIAN_POINT ( 'NONE',  ( 1.030449557444946671E-26, 53.50000000000031264, -24.09806918451526414 ) ) ;
#4136=LINE ( 'NONE', #6341, #8300 ) ;
#4138=CARTESIAN_POINT ( 'NONE',  ( 9.318419442923201951E-27, 47.50000000000033396, -26.00000000000011369 ) ) ;
#4139=LINE ( 'NONE', #4873, #955 ) ;
#4143=ADVANCED_FACE ( 'NONE', ( #3184 ), #6196, .F. ) ;
#4146=FACE_OUTER_BOUND ( 'NONE', #4839, .T. ) ;
#4158=VECTOR ( 'NONE', #1161, 1000.000000000000000 ) ;
#4160=VECTOR ( 'NONE', #6055, 1000.000000000000000 ) ;
#4166=CARTESIAN_POINT ( 'NONE',  ( -8.216777476527294510, 55.00000000000030553, -23.61111111111111427 ) ) ;
#4170=ORIENTED_EDGE ( 'NONE', *, *, #5490, .T. ) ;
#4171=DIRECTION ( 'NONE',  ( 1.820952055660014662E-28, 1.000000000000000000, 7.038118388768679669E-30 ) ) ;
#4172=ORIENTED_EDGE ( 'NONE', *, *, #7390, .F. ) ;
#4174=EDGE_LOOP ( 'NONE', ( #2011, #1833, #6874, #3858, #7895, #1839, #3316, #7750, #6, #7210, #240, #9293, #1690, #3321, #7267, #5504, #5486, #2470, #9189, #8823, #7772, #5270, #2050, #8670, #8940, #9434, #1706, #4842, #8990, #4954, #3480, #1423, #2650, #1298, #4093, #1150, #4698, #9453, #2769, #7424, #1852, #7239, #5957, #3606, #3671, #2331, #7618, #4286, #3125, #5157, #4696, #3784 ) ) ;
#4176=ADVANCED_FACE ( 'NONE', ( #382 ), #6484, .F. ) ;
#4183=ORIENTED_EDGE ( 'NONE', *, *, #6122, .T. ) ;
#4197=DIRECTION ( 'NONE',  ( 0.3286710990610922090, 6.289316826390952918E-29, 0.9444444444444435316 ) ) ;
#4222=PLANE ( 'NONE',  #4823 ) ;
#4230=DIRECTION ( 'NONE',  ( -0.3286710990610922090, -6.289316826390952918E-29, -0.9444444444444435316 ) ) ;
#4260=EDGE_CURVE ( 'NONE', #2949, #9099, #534, .T. ) ;
#4267=DIRECTION ( 'NONE',  ( -1.820952055660014662E-28, -1.000000000000000000, -7.038118388768679669E-30 ) ) ;
#4270=VERTEX_POINT ( 'NONE', #1314 ) ;
#4272=DIRECTION ( 'NONE',  ( 1.820952055660014662E-28, 1.000000000000000000, -6.508102468073347395E-30 ) ) ;
#4285=PLANE ( 'NONE',  #1340 ) ;
#4286=ORIENTED_EDGE ( 'NONE', *, *, #1715, .T. ) ;
#4288=CARTESIAN_POINT ( 'NONE',  ( 9.219811829770575476E-27, 46.00000000000018474, -24.09806918451533875 ) ) ;
#4289=ORIENTED_EDGE ( 'NONE', *, *, #5485, .T. ) ;
#4291=CARTESIAN_POINT ( 'NONE',  ( 8.677469957431129860E-27, 43.00000000000019895, -25.00000000000000000 ) ) ;
#4296=APPLICATION_CONTEXT ( 'automotive_design' ) ;
#4300=LINE ( 'NONE', #599, #1188 ) ;
#4309=ORIENTED_EDGE ( 'NONE', *, *, #6122, .F. ) ;
#4312=LINE ( 'NONE', #6520, #9073 ) ;
#4321=ADVANCED_FACE ( 'NONE', ( #4327 ), #7333, .F. ) ;
#4322=ORIENTED_EDGE ( 'NONE', *, *, #6251, .T. ) ;
#4323=DIRECTION ( 'NONE',  ( -1.820952055660014662E-28, -1.000000000000000000, -7.038118388768679669E-30 ) ) ;
#4327=FACE_OUTER_BOUND ( 'NONE', #3097, .T. ) ;
#4333=ADVANCED_FACE ( 'NONE', ( #4572 ), #7537, .F. ) ;
#4335=EDGE_CURVE ( 'NONE', #2857, #5882, #7479, .T. ) ;
#4341=FACE_OUTER_BOUND ( 'NONE', #8963, .T. ) ;
#4344=PLANE ( 'NONE',  #1916 ) ;
#4345=FACE_OUTER_BOUND ( 'NONE', #6126, .T. ) ;
#4347=CIRCLE ( 'NONE', #2434, 26.00000000000011369 ) ;
#4352=CARTESIAN_POINT ( 'NONE',  ( -8.216777476527294510, 43.00000000000019895, -23.61111111111111427 ) ) ;
#4356=LINE ( 'NONE', #3499, #1655 ) ;
#4363=ORIENTED_EDGE ( 'NONE', *, *, #937, .T. ) ;
#4368=AXIS2_PLACEMENT_3D ( 'NONE', #5718, #1325, #451 ) ;
#4376=CARTESIAN_POINT ( 'NONE',  ( 1.042775509089024980E-26, 52.00000000000031974, -26.00000000000006395 ) ) ;
#4381=DIRECTION ( 'NONE',  ( -1.820952055660014662E-28, -1.000000000000000000, -7.038118388768679669E-30 ) ) ;
#4384=CARTESIAN_POINT ( 'NONE',  ( 1.138917931912835794E-26, 58.00000000000029132, -25.00000000000000000 ) ) ;
#4392=CARTESIAN_POINT ( 'NONE',  ( 5.423418723394456162E-28, -2.066522830327504070E-28, -26.00000000000014566 ) ) ;
#4394=LINE ( 'NONE', #7396, #3357 ) ;
#4395=DIRECTION ( 'NONE',  ( -0.1666666666666658525, -3.897465909857536228E-29, -0.9860132971832695770 ) ) ;
#4403=DIRECTION ( 'NONE',  ( 0.9860132971832693549, 1.788557213313974126E-28, -0.1666666666666657970 ) ) ;
#4409=CARTESIAN_POINT ( 'NONE',  ( 9.762153702110021092E-27, 50.50000000000031974, -25.00000000000000000 ) ) ;
#4411=CARTESIAN_POINT ( 'NONE',  ( -8.545448575588423523, -1.752403656397945903E-27, -24.55555555555572766 ) ) ;
#4414=AXIS2_PLACEMENT_3D ( 'NONE', #6628, #3626, #8217 ) ;
#4421=FACE_OUTER_BOUND ( 'NONE', #8513, .T. ) ;
#4435=DIRECTION ( 'NONE',  ( 0.9444444444444436426, 1.704463408222248963E-28, -0.3286710990610922645 ) ) ;
#4436=PLANE ( 'NONE',  #653 ) ;
#4451=EDGE_CURVE ( 'NONE', #6620, #7071, #1556, .T. ) ;
#4452=CARTESIAN_POINT ( 'NONE',  ( 1.094544505994153880E-26, 56.50000000000029843, -25.00000000000000000 ) ) ;
#4459=ORIENTED_EDGE ( 'NONE', *, *, #7023, .T. ) ;
#4462=CARTESIAN_POINT ( 'NONE',  ( 9.196165333680795946E-27, 50.50000000000031974, 3.170080688461390214E-28 ) ) ;
#4467=CARTESIAN_POINT ( 'NONE',  ( 1.047999611769018552E-26, 57.50000000000029843, 3.031413732465509233E-28 ) ) ;
#4474=EDGE_CURVE ( 'NONE', #5419, #3082, #2177, .T. ) ;
#4477=PLANE ( 'NONE',  #250 ) ;
#4492=EDGE_CURVE ( 'NONE', #9092, #3225, #5578, .T. ) ;
#4499=CARTESIAN_POINT ( 'NONE',  ( -0.1666666666666679342, 60.00000000000029843, -25.98601329718323782 ) ) ;
#4503=AXIS2_PLACEMENT_3D ( 'NONE', #2316, #6713, #947 ) ;
#4505=AXIS2_PLACEMENT_3D ( 'NONE', #4467, #8166, #1397 ) ;
#4521=LINE ( 'NONE', #616, #6972 ) ;
#4529=DIRECTION ( 'NONE',  ( -1.820952055660014662E-28, -1.000000000000000000, -7.038118388768679669E-30 ) ) ;
#4540=LINE ( 'NONE', #6787, #5161 ) ;
#4561=CARTESIAN_POINT ( 'NONE',  ( -8.216777476527294510, 57.50000000000029843, -23.61111111111111427 ) ) ;
#4563=EDGE_CURVE ( 'NONE', #3415, #7610, #1455, .T. ) ;
#4566=VECTOR ( 'NONE', #580, 1000.000000000000000 ) ;
#4569=VERTEX_POINT ( 'NONE', #4133 ) ;
#4572=FACE_OUTER_BOUND ( 'NONE', #6301, .T. ) ;
#4578=PRODUCT_DEFINITION_SHAPE ( 'NONE', 'NONE',  #8871 ) ;
#4586=DIRECTION ( 'NONE',  ( -1.820952055660014662E-28, -1.000000000000000000, -7.038118388768679669E-30 ) ) ;
#4589=DIRECTION ( 'NONE',  ( 1.735493991486225972E-29, -6.508102468073347395E-30, -1.000000000000000000 ) ) ;
#4614=CARTESIAN_POINT ( 'NONE',  ( -12.16083066526041989, 40.00000000000014921, -34.94444444444444287 ) ) ;
#4624=ORIENTED_EDGE ( 'NONE', *, *, #6232, .T. ) ;
#4652=CIRCLE ( 'NONE', #2266, 26.00000000000004974 ) ;
#4660=ORIENTED_EDGE ( 'NONE', *, *, #5889, .T. ) ;
#4668=LINE ( 'NONE', #4020, #7978 ) ;
#4679=VECTOR ( 'NONE', #5053, 1000.000000000000000 ) ;
#4687=CARTESIAN_POINT ( 'NONE',  ( -8.216777476527294510, 56.00000000000030553, -23.61111111111111427 ) ) ;
#4693=EDGE_CURVE ( 'NONE', #2443, #5928, #8925, .T. ) ;
#4696=ORIENTED_EDGE ( 'NONE', *, *, #5051, .T. ) ;
#4697=DIRECTION ( 'NONE',  ( 1.735493991486227373E-29, 0.000000000000000000, -1.000000000000000000 ) ) ;
#4698=ORIENTED_EDGE ( 'NONE', *, *, #2373, .T. ) ;
#4700=CARTESIAN_POINT ( 'NONE',  ( 1.040310318760209318E-26, 47.50000000000033396, -25.00000000000000000 ) ) ;
#4712=ORIENTED_EDGE ( 'NONE', *, *, #6721, .F. ) ;
#4718=FACE_OUTER_BOUND ( 'NONE', #6328, .T. ) ;
#4728=( NAMED_UNIT ( * ) PLANE_ANGLE_UNIT ( ) SI_UNIT ( $, .RADIAN. ) );
#4735=VECTOR ( 'NONE', #8629, 1000.000000000000341 ) ;
#4742=ORIENTED_EDGE ( 'NONE', *, *, #5995, .T. ) ;
#4743=EDGE_CURVE ( 'NONE', #185, #2421, #3126, .T. ) ;
#4755=EDGE_LOOP ( 'NONE', ( #1153, #5150, #2065, #2776 ) ) ;
#4760=CARTESIAN_POINT ( 'NONE',  ( 5.423418723394456162E-28, -2.066522830327504070E-28, -26.00000000000003197 ) ) ;
#4776=LINE ( 'NONE', #7782, #4735 ) ;
#4778=FACE_OUTER_BOUND ( 'NONE', #4860, .T. ) ;
#4785=VECTOR ( 'NONE', #1212, 1000.000000000000000 ) ;
#4799=VERTEX_POINT ( 'NONE', #2386 ) ;
#4805=VECTOR ( 'NONE', #785, 1000.000000000000000 ) ;
#4806=LINE ( 'NONE', #4166, #8397 ) ;
#4807=DIRECTION ( 'NONE',  ( -1.735493991486225972E-29, 6.508102468073347395E-30, 1.000000000000000000 ) ) ;
#4809=VECTOR ( 'NONE', #9111, 1000.000000000000000 ) ;
#4821=DIRECTION ( 'NONE',  ( -1.735493991486225972E-29, 6.508102468073347395E-30, 1.000000000000000000 ) ) ;
#4823=AXIS2_PLACEMENT_3D ( 'NONE', #8059, #7217, #5047 ) ;
#4826=VECTOR ( 'NONE', #829, 1000.000000000000000 ) ;
#4830=CARTESIAN_POINT ( 'NONE',  ( -8.545448575588382667, 47.50000000000033396, -24.55555555555566372 ) ) ;
#4835=AXIS2_PLACEMENT_3D ( 'NONE', #8404, #5295, #2313 ) ;
#4838=PLANE ( 'NONE',  #708 ) ;
#4839=EDGE_LOOP ( 'NONE', ( #8018, #9151, #3757, #945 ) ) ;
#4842=ORIENTED_EDGE ( 'NONE', *, *, #1181, .T. ) ;
#4858=ORIENTED_EDGE ( 'NONE', *, *, #7049, .T. ) ;
#4859=CYLINDRICAL_SURFACE ( 'NONE', #571, 26.00000000000006395 ) ;
#4860=EDGE_LOOP ( 'NONE', ( #6546, #7292, #4624, #473 ) ) ;
#4867=DIRECTION ( 'NONE',  ( 1.820952055660014662E-28, 1.000000000000000000, -6.508102468073347395E-30 ) ) ;
#4869=DIRECTION ( 'NONE',  ( 1.735493991486225972E-29, -6.508102468073347395E-30, -1.000000000000000000 ) ) ;
#4873=CARTESIAN_POINT ( 'NONE',  ( 1.084683744678891232E-26, 48.50000000000033396, -37.00000000000000711 ) ) ;
#4882=LINE ( 'NONE', #4291, #274 ) ;
#4915=ADVANCED_FACE ( 'NONE', ( #3273 ), #7929, .F. ) ;
#4920=EDGE_CURVE ( 'NONE', #9740, #3225, #8572, .T. ) ;
#4928=EDGE_CURVE ( 'NONE', #1931, #3415, #4776, .T. ) ;
#4931=LINE ( 'NONE', #7944, #2361 ) ;
#4933=EDGE_CURVE ( 'NONE', #7524, #6996, #3327, .T. ) ;
#4935=DIRECTION ( 'NONE',  ( -1.820952055660014662E-28, -1.000000000000000000, 6.508102468073347395E-30 ) ) ;
#4940=VECTOR ( 'NONE', #8262, 1000.000000000000000 ) ;
#4943=EDGE_LOOP ( 'NONE', ( #8370, #3398, #1347, #3435 ) ) ;
#4946=ORIENTED_EDGE ( 'NONE', *, *, #2373, .F. ) ;
#4949=FACE_OUTER_BOUND ( 'NONE', #956, .T. ) ;
#4953=CARTESIAN_POINT ( 'NONE',  ( -8.216777476527274970, 78.08723716182652197, -23.61111111111111427 ) ) ;
#4954=ORIENTED_EDGE ( 'NONE', *, *, #1633, .F. ) ;
#4959=VECTOR ( 'NONE', #6585, 1000.000000000000000 ) ;
#4961=CARTESIAN_POINT ( 'NONE',  ( 1.555535097482682654E-26, 78.08723716182652197, -25.00000000000000000 ) ) ;
#4963=ORIENTED_EDGE ( 'NONE', *, *, #8365, .T. ) ;
#4972=CARTESIAN_POINT ( 'NONE',  ( 9.389914726526274261E-27, 51.50000000000032685, 2.896598636358402723E-28 ) ) ;
#4974=VECTOR ( 'NONE', #2025, 1000.000000000000000 ) ;
#4980=ORIENTED_EDGE ( 'NONE', *, *, #965, .T. ) ;
#4982=DIRECTION ( 'NONE',  ( 1.735493991486225972E-29, -6.508102468073347395E-30, -1.000000000000000000 ) ) ;
#4988=LINE ( 'NONE', #724, #3669 ) ;
#4993=ORIENTED_EDGE ( 'NONE', *, *, #710, .F. ) ;
#4994=DIRECTION ( 'NONE',  ( -1.735493991486225972E-29, 6.508102468073347395E-30, 1.000000000000000000 ) ) ;
#5007=ORIENTED_EDGE ( 'NONE', *, *, #7272, .T. ) ;
#5009=ORIENTED_EDGE ( 'NONE', *, *, #255, .F. ) ;
#5017=LINE ( 'NONE', #8123, #1799 ) ;
#5032=CARTESIAN_POINT ( 'NONE',  ( 1.555535097482682654E-26, 78.08723716182652197, -25.00000000000000000 ) ) ;
#5033=ADVANCED_FACE ( 'NONE', ( #3939 ), #9131, .F. ) ;
#5034=ORIENTED_EDGE ( 'NONE', *, *, #4068, .F. ) ;
#5042=CARTESIAN_POINT ( 'NONE',  ( 1.040310318760209318E-26, 55.00000000000030553, -26.00000000000003197 ) ) ;
#5043=DIRECTION ( 'NONE',  ( 1.735493991486225972E-29, -6.508102468073347395E-30, -1.000000000000000000 ) ) ;
#5047=DIRECTION ( 'NONE',  ( -0.9860132971832694659, -1.788557213313974350E-28, 0.1666666666666658247 ) ) ;
#5051=EDGE_CURVE ( 'NONE', #3045, #2848, #8385, .T. ) ;
#5053=DIRECTION ( 'NONE',  ( -1.820952055660014662E-28, -1.000000000000000000, -7.038118388768679669E-30 ) ) ;
#5055=ORIENTED_EDGE ( 'NONE', *, *, #930, .T. ) ;
#5056=EDGE_CURVE ( 'NONE', #269, #2192, #1904, .T. ) ;
#5064=CARTESIAN_POINT ( 'NONE',  ( 9.661664702339496822E-27, 53.00000000000031974, 2.823413298471687761E-28 ) ) ;
#5069=CARTESIAN_POINT ( 'NONE',  ( -8.216777476527294510, 54.50000000000031264, -23.61111111111111427 ) ) ;
#5071=VECTOR ( 'NONE', #3786, 1000.000000000000000 ) ;
#5076=ORIENTED_EDGE ( 'NONE', *, *, #2329, .F. ) ;
#5099=ORIENTED_EDGE ( 'NONE', *, *, #4451, .T. ) ;
#5114=CARTESIAN_POINT ( 'NONE',  ( 8.106083942516887559E-27, 44.50000000000019185, 2.954376534690019799E-28 ) ) ;
#5122=VECTOR ( 'NONE', #3136, 1000.000000000000000 ) ;
#5126=CARTESIAN_POINT ( 'NONE',  ( 1.097009696322969542E-26, 52.00000000000031974, -25.00000000000000000 ) ) ;
#5133=PLANE ( 'NONE',  #319 ) ;
#5135=CIRCLE ( 'NONE', #5459, 26.00000000000015987 ) ;
#5143=LINE ( 'NONE', #8195, #1293 ) ;
#5145=AXIS2_PLACEMENT_3D ( 'NONE', #6809, #2205, #3006 ) ;
#5150=ORIENTED_EDGE ( 'NONE', *, *, #8819, .T. ) ;
#5155=ORIENTED_EDGE ( 'NONE', *, *, #2926, .T. ) ;
#5157=ORIENTED_EDGE ( 'NONE', *, *, #7514, .F. ) ;
#5161=VECTOR ( 'NONE', #3742, 1000.000000000000000 ) ;
#5168=DIRECTION ( 'NONE',  ( 1.000000000000000000, 0.000000000000000000, 0.000000000000000000 ) ) ;
#5171=CARTESIAN_POINT ( 'NONE',  ( 9.922629470464150863E-27, 54.50000000000031264, 2.962080254467568742E-28 ) ) ;
#5184=DIRECTION ( 'NONE',  ( -0.3286710990610922090, -6.289316826390952918E-29, -0.9444444444444435316 ) ) ;
#5189=FACE_OUTER_BOUND ( 'NONE', #8033, .T. ) ;
#5193=SHAPE_DEFINITION_REPRESENTATION ( #4578, #1483 ) ;
#5199=CARTESIAN_POINT ( 'NONE',  ( -12.16083066526040213, 60.00000000000029843, -34.94444444444452103 ) ) ;
#5203=CARTESIAN_POINT ( 'NONE',  ( 9.417027056075828427E-27, 44.50000000000019185, -25.00000000000000000 ) ) ;
#5208=VERTEX_POINT ( 'NONE', #1756 ) ;
#5221=DIRECTION ( 'NONE',  ( -1.820952055660014662E-28, -1.000000000000000000, -7.038118388768679669E-30 ) ) ;
#5223=DIRECTION ( 'NONE',  ( -1.820952055660014662E-28, -1.000000000000000000, -7.038118388768679669E-30 ) ) ;
#5227=EDGE_CURVE ( 'NONE', #9622, #9126, #4139, .T. ) ;
#5228=FACE_OUTER_BOUND ( 'NONE', #5450, .T. ) ;
#5232=CARTESIAN_POINT ( 'NONE',  ( 1.153709073885729765E-26, 55.00000000000030553, -37.00000000000000711 ) ) ;
#5235=DIRECTION ( 'NONE',  ( -0.9860132971832693549, -1.788557213313974126E-28, 0.1666666666666657970 ) ) ;
#5236=LINE ( 'NONE', #648, #8921 ) ;
#5237=CYLINDRICAL_SURFACE ( 'NONE', #3302, 26.00000000000008171 ) ;
#5244=DIRECTION ( 'NONE',  ( -0.9860132971832693549, -1.788449361237088441E-28, 0.1666666666666662133 ) ) ;
#5248=LINE ( 'NONE', #8259, #4809 ) ;
#5251=LINE ( 'NONE', #6579, #4940 ) ;
#5255=DIRECTION ( 'NONE',  ( 0.3286710990610922090, 6.289316826390952918E-29, 0.9444444444444435316 ) ) ;
#5270=ORIENTED_EDGE ( 'NONE', *, *, #5485, .F. ) ;
#5271=ADVANCED_FACE ( 'NONE', ( #3386 ), #1451, .F. ) ;
#5277=ORIENTED_EDGE ( 'NONE', *, *, #1848, .F. ) ;
#5284=EDGE_CURVE ( 'NONE', #8065, #3045, #7480, .T. ) ;
#5295=DIRECTION ( 'NONE',  ( -1.820952055660014662E-28, -1.000000000000000000, 6.508102468073347395E-30 ) ) ;
#5299=DIRECTION ( 'NONE',  ( 0.9860132971832693549, 1.788557213313974126E-28, -0.1666666666666657970 ) ) ;
#5308=CARTESIAN_POINT ( 'NONE',  ( 1.138917931912835794E-26, 58.00000000000029132, -25.00000000000000000 ) ) ;
#5323=CARTESIAN_POINT ( 'NONE',  ( -8.216777476527294510, 44.50000000000019185, -23.61111111111111427 ) ) ;
#5325=FACE_OUTER_BOUND ( 'NONE', #4174, .T. ) ;
#5329=LINE ( 'NONE', #3843, #5122 ) ;
#5331=ORIENTED_EDGE ( 'NONE', *, *, #2685, .F. ) ;
#5338=CARTESIAN_POINT ( 'NONE',  ( -8.216777476527274970, 78.08723716182652197, -23.61111111111111427 ) ) ;
#5343=LINE ( 'NONE', #3809, #1038 ) ;
#5348=PLANE ( 'NONE',  #8615 ) ;
#5350=EDGE_CURVE ( 'NONE', #4048, #7113, #4119, .T. ) ;
#5352=LINE ( 'NONE', #8409, #8294 ) ;
#5357=CARTESIAN_POINT ( 'NONE',  ( -8.545448575588403983, 42.50000000000020606, -24.55555555555568858 ) ) ;
#5359=EDGE_LOOP ( 'NONE', ( #3715, #3814, #3748, #6623 ) ) ;
#5364=AXIS2_PLACEMENT_3D ( 'NONE', #488, #2045, #6399 ) ;
#5371=ORIENTED_EDGE ( 'NONE', *, *, #6106, .T. ) ;
#5375=CARTESIAN_POINT ( 'NONE',  ( 1.555535097482682654E-26, 78.08723716182652197, -25.00000000000000000 ) ) ;
#5382=CARTESIAN_POINT ( 'NONE',  ( 1.040310318760209318E-26, 50.00000000000032685, -26.00000000000009592 ) ) ;
#5397=VERTEX_POINT ( 'NONE', #3627 ) ;
#5399=VECTOR ( 'NONE', #2051, 1000.000000000000000 ) ;
#5404=VECTOR ( 'NONE', #1146, 1000.000000000000000 ) ;
#5407=DIRECTION ( 'NONE',  ( 1.735493991486225972E-29, -6.508102468073347395E-30, -1.000000000000000000 ) ) ;
#5410=DIRECTION ( 'NONE',  ( 1.735493991486225972E-29, -6.508102468073347395E-30, -1.000000000000000000 ) ) ;
#5415=ADVANCED_FACE ( 'NONE', ( #8270 ), #9013, .F. ) ;
#5419=VERTEX_POINT ( 'NONE', #232 ) ;
#5423=ORIENTED_EDGE ( 'NONE', *, *, #6106, .F. ) ;
#5430=DIRECTION ( 'NONE',  ( -1.820952055660014662E-28, -1.000000000000000000, -7.038118388768679669E-30 ) ) ;
#5432=CARTESIAN_POINT ( 'NONE',  ( 1.148778693228098442E-26, 57.50000000000029843, -25.00000000000000000 ) ) ;
#5442=ADVANCED_FACE ( 'NONE', ( #3882 ), #3021, .F. ) ;
#5446=FACE_OUTER_BOUND ( 'NONE', #8318, .T. ) ;
#5449=VECTOR ( 'NONE', #6411, 1000.000000000000000 ) ;
#5450=EDGE_LOOP ( 'NONE', ( #5034, #8551, #8438, #3999 ) ) ;
#5457=VECTOR ( 'NONE', #8702, 1000.000000000000000 ) ;
#5459=AXIS2_PLACEMENT_3D ( 'NONE', #2070, #5876, #6518 ) ;
#5460=VECTOR ( 'NONE', #8139, 1000.000000000000000 ) ;
#5468=ORIENTED_EDGE ( 'NONE', *, *, #5995, .F. ) ;
#5472=EDGE_LOOP ( 'NONE', ( #7678, #6189, #7255, #4070 ) ) ;
#5483=VECTOR ( 'NONE', #3634, 1000.000000000000000 ) ;
#5484=PLANE ( 'NONE',  #1642 ) ;
#5485=EDGE_CURVE ( 'NONE', #2731, #5636, #9547, .T. ) ;
#5486=ORIENTED_EDGE ( 'NONE', *, *, #3461, .T. ) ;
#5490=EDGE_CURVE ( 'NONE', #5397, #3415, #5248, .T. ) ;
#5504=ORIENTED_EDGE ( 'NONE', *, *, #163, .T. ) ;
#5510=DIRECTION ( 'NONE',  ( -0.1666666666666658525, -3.897465909857536228E-29, -0.9860132971832695770 ) ) ;
#5518=CARTESIAN_POINT ( 'NONE',  ( -8.216777476527294510, 58.00000000000029132, -23.61111111111107519 ) ) ;
#5528=ORIENTED_EDGE ( 'NONE', *, *, #8060, .F. ) ;
#5546=LINE ( 'NONE', #7058, #7085 ) ;
#5547=ORIENTED_EDGE ( 'NONE', *, *, #2925, .T. ) ;
#5555=CARTESIAN_POINT ( 'NONE',  ( 1.099474886651785204E-26, 56.50000000000029843, -37.00000000000000711 ) ) ;
#5566=VECTOR ( 'NONE', #75, 1000.000000000000000 ) ;
#5570=CARTESIAN_POINT ( 'NONE',  ( 1.028855784077797189E-26, 56.50000000000029843, 3.062228611575705006E-28 ) ) ;
#5578=LINE ( 'NONE', #6211, #8516 ) ;
#5582=ORIENTED_EDGE ( 'NONE', *, *, #586, .T. ) ;
#5583=CARTESIAN_POINT ( 'NONE',  ( -8.545448575588384443, 52.00000000000031974, -24.55555555555561753 ) ) ;
#5584=LINE ( 'NONE', #6268, #3091 ) ;
#5589=DIRECTION ( 'NONE',  ( 1.735493991486225972E-29, -6.508102468073347395E-30, -1.000000000000000000 ) ) ;
#5592=VERTEX_POINT ( 'NONE', #18 ) ;
#5593=CARTESIAN_POINT ( 'NONE',  ( 9.318419442923201951E-27, 49.00000000000032685, -26.00000000000009592 ) ) ;
#5608=CARTESIAN_POINT ( 'NONE',  ( 9.762153702110021092E-27, 48.50000000000033396, -24.09806918451532809 ) ) ;
#5610=AXIS2_PLACEMENT_3D ( 'NONE', #1794, #3324, #3431 ) ;
#5612=CARTESIAN_POINT ( 'NONE',  ( 0.000000000000000000, 0.000000000000000000, 0.000000000000000000 ) ) ;
#5613=DIRECTION ( 'NONE',  ( 1.735493991486225972E-29, -6.508102468073347395E-30, -1.000000000000000000 ) ) ;
#5617=LINE ( 'NONE', #1858, #5753 ) ;
#5631=AXIS2_PLACEMENT_3D ( 'NONE', #3087, #7397, #4589 ) ;
#5632=LINE ( 'NONE', #7861, #9252 ) ;
#5636=VERTEX_POINT ( 'NONE', #1082 ) ;
#5638=VERTEX_POINT ( 'NONE', #6450 ) ;
#5640=ADVANCED_FACE ( 'NONE', ( #5772 ), #395, .F. ) ;
#5661=PLANE ( 'NONE',  #8068 ) ;
#5667=DIRECTION ( 'NONE',  ( 1.820952055660014662E-28, 1.000000000000000000, 7.038118388768679669E-30 ) ) ;
#5681=DIRECTION ( 'NONE',  ( 1.735493991486226532E-29, 0.000000000000000000, -1.000000000000000000 ) ) ;
#5691=ORIENTED_EDGE ( 'NONE', *, *, #9460, .T. ) ;
#5702=ORIENTED_EDGE ( 'NONE', *, *, #9582, .F. ) ;
#5703=LINE ( 'NONE', #482, #4959 ) ;
#5707=LINE ( 'NONE', #9511, #1281 ) ;
#5717=CARTESIAN_POINT ( 'NONE',  ( 5.423418723394456162E-28, -2.066522830327504070E-28, -26.00000000000004974 ) ) ;
#5718=CARTESIAN_POINT ( 'NONE',  ( 1.636886378333599496E-26, 78.08723716182652197, -37.00000000000000711 ) ) ;
#5719=EDGE_CURVE ( 'NONE', #9428, #2716, #5860, .T. ) ;
#5721=VECTOR ( 'NONE', #8042, 1000.000000000000000 ) ;
#5722=DIRECTION ( 'NONE',  ( 1.735493991486225972E-29, -6.508102468073347395E-30, -1.000000000000000000 ) ) ;
#5730=VERTEX_POINT ( 'NONE', #9753 ) ;
#5731=CARTESIAN_POINT ( 'NONE',  ( 8.677469957431129860E-27, 45.50000000000019185, -26.00000000000014566 ) ) ;
#5732=LINE ( 'NONE', #2564, #8288 ) ;
#5735=DIRECTION ( 'NONE',  ( 1.735493991486225972E-29, -6.508102468073347395E-30, -1.000000000000000000 ) ) ;
#5736=ORIENTED_EDGE ( 'NONE', *, *, #8975, .F. ) ;
#5744=CARTESIAN_POINT ( 'NONE',  ( -8.545448575588393325, 44.50000000000019185, -24.55555555555569569 ) ) ;
#5753=VECTOR ( 'NONE', #7285, 1000.000000000000000 ) ;
#5763=ORIENTED_EDGE ( 'NONE', *, *, #2487, .T. ) ;
#5767=AXIS2_PLACEMENT_3D ( 'NONE', #9395, #4067, #4807 ) ;
#5769=CARTESIAN_POINT ( 'NONE',  ( -8.216777476527294510, 53.50000000000031264, -23.61111111111107519 ) ) ;
#5772=FACE_OUTER_BOUND ( 'NONE', #4755, .T. ) ;
#5782=LINE ( 'NONE', #6455, #6975 ) ;
#5784=ORIENTED_EDGE ( 'NONE', *, *, #574, .F. ) ;
#5794=ORIENTED_EDGE ( 'NONE', *, *, #107, .F. ) ;
#5799=LINE ( 'NONE', #5840, #532 ) ;
#5808=APPLICATION_CONTEXT ( 'automotive_design' ) ;
#5817=CARTESIAN_POINT ( 'NONE',  ( -8.216777476527294510, 50.00000000000032685, -23.61111111111111427 ) ) ;
#5820=ORIENTED_EDGE ( 'NONE', *, *, #4492, .T. ) ;
#5821=LINE ( 'NONE', #2059, #683 ) ;
#5828=AXIS2_PLACEMENT_3D ( 'NONE', #3796, #9086, #2302 ) ;
#5840=CARTESIAN_POINT ( 'NONE',  ( 9.762153702110021092E-27, 50.50000000000031974, -25.00000000000000000 ) ) ;
#5846=CARTESIAN_POINT ( 'NONE',  ( -8.545448575588375562, 55.00000000000030553, -24.55555555555558911 ) ) ;
#5848=STYLED_ITEM('',(#9806),#9647);
#5850=DIRECTION ( 'NONE',  ( -1.820952055660014662E-28, -1.000000000000000000, -7.038118388768679669E-30 ) ) ;
#5852=VECTOR ( 'NONE', #6783, 1000.000000000000000 ) ;
#5856=DIRECTION ( 'NONE',  ( -1.820952055660014662E-28, -1.000000000000000000, 6.508102468073347395E-30 ) ) ;
#5858=DIRECTION ( 'NONE',  ( 1.735493991486225972E-29, -6.508102468073347395E-30, -1.000000000000000000 ) ) ;
#5860=LINE ( 'NONE', #3595, #7964 ) ;
#5871=VECTOR ( 'NONE', #8906, 1000.000000000000000 ) ;
#5872=VECTOR ( 'NONE', #2401, 1000.000000000000000 ) ;
#5876=DIRECTION ( 'NONE',  ( -1.820952055660014662E-28, -1.000000000000000000, -7.038118388768679669E-30 ) ) ;
#5879=CARTESIAN_POINT ( 'NONE',  ( 1.138917931912835794E-26, 56.00000000000030553, -25.00000000000000000 ) ) ;
#5882=VERTEX_POINT ( 'NONE', #3237 ) ;
#5885=DIRECTION ( 'NONE',  ( 0.3286710990610922090, 6.289316826390952918E-29, 0.9444444444444435316 ) ) ;
#5886=ADVANCED_FACE ( 'NONE', ( #149 ), #1621, .F. ) ;
#5889=EDGE_CURVE ( 'NONE', #9126, #9742, #5329, .T. ) ;
#5893=DIRECTION ( 'NONE',  ( -1.820952055660014662E-28, -1.000000000000000000, 6.508102468073347395E-30 ) ) ;
#5908=VECTOR ( 'NONE', #3678, 1000.000000000000341 ) ;
#5910=DIRECTION ( 'NONE',  ( 0.9860132971832693549, 1.788557213313974126E-28, -0.1666666666666657970 ) ) ;
#5928=VERTEX_POINT ( 'NONE', #6151 ) ;
#5931=FACE_OUTER_BOUND ( 'NONE', #9348, .T. ) ;
#5937=LINE ( 'NONE', #5976, #3355 ) ;
#5942=CARTESIAN_POINT ( 'NONE',  ( 1.257247067695987565E-26, 60.00000000000029843, -37.00000000000000711 ) ) ;
#5943=( NAMED_UNIT ( * ) PLANE_ANGLE_UNIT ( ) SI_UNIT ( $, .RADIAN. ) );
#5956=DIRECTION ( 'NONE',  ( 1.735493991486225692E-29, -6.508102468073347395E-30, -1.000000000000000000 ) ) ;
#5957=ORIENTED_EDGE ( 'NONE', *, *, #6948, .T. ) ;
#5960=VERTEX_POINT ( 'NONE', #2345 ) ;
#5961=DIRECTION ( 'NONE',  ( 0.9860132971832693549, 1.788557213313974126E-28, -0.1666666666666657970 ) ) ;
#5976=CARTESIAN_POINT ( 'NONE',  ( 5.423418723394456162E-28, -2.066522830327504070E-28, -26.00000000000006395 ) ) ;
#5984=SHAPE_REPRESENTATION_RELATIONSHIP ( 'NONE' , 'NONE' ,  #1483, #1270 ) ;
#5986=LINE ( 'NONE', #7437, #5908 ) ;
#5987=AXIS2_PLACEMENT_3D ( 'NONE', #3035, #973, #2442 ) ;
#5990=EDGE_CURVE ( 'NONE', #3624, #1910, #7696, .T. ) ;
#5991=EDGE_CURVE ( 'NONE', #2117, #8507, #929, .T. ) ;
#5994=CARTESIAN_POINT ( 'NONE',  ( -8.216777476527294510, 46.00000000000018474, -23.61111111111111427 ) ) ;
#5995=EDGE_CURVE ( 'NONE', #1637, #5928, #248, .T. ) ;
#6009=CARTESIAN_POINT ( 'NONE',  ( 8.369359826574806283E-27, 46.00000000000018474, 2.927413515468598497E-28 ) ) ;
#6019=CARTESIAN_POINT ( 'NONE',  ( 1.084683744678891232E-26, 56.00000000000030553, -24.09806918451524638 ) ) ;
#6020=ORIENTED_EDGE ( 'NONE', *, *, #2441, .T. ) ;
#6031=VERTEX_POINT ( 'NONE', #7848 ) ;
#6033=CARTESIAN_POINT ( 'NONE',  ( 7.592786212752238627E-27, 43.00000000000019895, -24.09806918451537072 ) ) ;
#6042=LINE ( 'NONE', #7550, #336 ) ;
#6043=VECTOR ( 'NONE', #7853, 1000.000000000000000 ) ;
#6048=AXIS2_PLACEMENT_3D ( 'NONE', #6200, #1666, #9182 ) ;
#6055=DIRECTION ( 'NONE',  ( 0.3286710990610922090, 6.289316826390952918E-29, 0.9444444444444435316 ) ) ;
#6060=ADVANCED_FACE ( 'NONE', ( #445 ), #4285, .F. ) ;
#6068=VECTOR ( 'NONE', #5735, 1000.000000000000000 ) ;
#6073=PLANE ( 'NONE',  #4835 ) ;
#6078=ORIENTED_EDGE ( 'NONE', *, *, #7518, .T. ) ;
#6086=ORIENTED_EDGE ( 'NONE', *, *, #6951, .T. ) ;
#6088=CLOSED_SHELL ( 'NONE', ( #2179, #4333, #5886, #4143, #164, #9626, #5640, #6060, #1656, #6294, #217, #9658, #9447, #8235, #3909, #2418, #793, #4321, #6357, #4176, #5415, #1271, #2439, #9524, #8912, #8215, #2497, #5033, #6464, #9579, #771, #4915, #524, #2974, #6597, #9509, #1127, #150, #3848, #2797, #8389, #770, #8969, #762, #1837, #5442, #9017, #3778, #2242, #6246, #6722, #5271, #7150, #6492 ) ) ;
#6091=ORIENTED_EDGE ( 'NONE', *, *, #1672, .F. ) ;
#6093=DIRECTION ( 'NONE',  ( 1.735493991486225972E-29, -6.508102468073347395E-30, -1.000000000000000000 ) ) ;
#6106=EDGE_CURVE ( 'NONE', #3950, #77, #5617, .T. ) ;
#6107=CARTESIAN_POINT ( 'NONE',  ( -8.216777476527294510, 44.00000000000019895, -23.61111111111111427 ) ) ;
#6112=CARTESIAN_POINT ( 'NONE',  ( 9.417027056075828427E-27, 44.50000000000019185, -25.00000000000000000 ) ) ;
#6121=DIRECTION ( 'NONE',  ( 1.735493991486227934E-29, 0.000000000000000000, -1.000000000000000000 ) ) ;
#6122=EDGE_CURVE ( 'NONE', #2716, #7071, #8276, .T. ) ;
#6126=EDGE_LOOP ( 'NONE', ( #1329, #5794, #7472, #5528 ) ) ;
#6135=DIRECTION ( 'NONE',  ( -1.820952055660014662E-28, -1.000000000000000000, -7.038118388768679669E-30 ) ) ;
#6143=LINE ( 'NONE', #9176, #5071 ) ;
#6151=CARTESIAN_POINT ( 'NONE',  ( 8.677469957431129860E-27, 40.00000000000014921, -25.00000000000000000 ) ) ;
#6155=CARTESIAN_POINT ( 'NONE',  ( -8.216777476527294510, 40.00000000000014921, -23.61111111111111427 ) ) ;
#6156=VERTEX_POINT ( 'NONE', #5069 ) ;
#6159=ORIENTED_EDGE ( 'NONE', *, *, #6951, .F. ) ;
#6165=EDGE_LOOP ( 'NONE', ( #8717, #8003, #7613, #318 ) ) ;
#6172=LINE ( 'NONE', #7717, #5566 ) ;
#6177=ORIENTED_EDGE ( 'NONE', *, *, #3476, .T. ) ;
#6189=ORIENTED_EDGE ( 'NONE', *, *, #7940, .F. ) ;
#6193=ORIENTED_EDGE ( 'NONE', *, *, #1407, .T. ) ;
#6196=PLANE ( 'NONE',  #2033 ) ;
#6199=EDGE_LOOP ( 'NONE', ( #5736, #3541, #3727, #1873 ) ) ;
#6200=CARTESIAN_POINT ( 'NONE',  ( 1.555535097482682654E-26, 78.08723716182652197, -25.00000000000000000 ) ) ;
#6208=CIRCLE ( 'NONE', #8581, 26.00000000000002132 ) ;
#6210=ORIENTED_EDGE ( 'NONE', *, *, #2329, .T. ) ;
#6211=CARTESIAN_POINT ( 'NONE',  ( -8.216777476527294510, 60.00000000000029843, -23.61111111111107519 ) ) ;
#6231=VECTOR ( 'NONE', #2874, 1000.000000000000000 ) ;
#6232=EDGE_CURVE ( 'NONE', #1238, #8006, #721, .T. ) ;
#6234=VECTOR ( 'NONE', #6635, 1000.000000000000000 ) ;
#6243=EDGE_LOOP ( 'NONE', ( #9545, #8355, #7311, #8471 ) ) ;
#6246=ADVANCED_FACE ( 'NONE', ( #6539 ), #4477, .F. ) ;
#6251=EDGE_CURVE ( 'NONE', #6987, #3873, #5986, .T. ) ;
#6268=CARTESIAN_POINT ( 'NONE',  ( 1.148778693228098442E-26, 57.50000000000029843, -25.00000000000000000 ) ) ;
#6274=DIRECTION ( 'NONE',  ( -0.9860132971832693549, -1.788557213313974126E-28, 0.1666666666666657970 ) ) ;
#6285=CARTESIAN_POINT ( 'NONE',  ( -12.16083066526040213, 78.08723716182652197, -34.94444444444459918 ) ) ;
#6294=ADVANCED_FACE ( 'NONE', ( #4718 ), #918, .F. ) ;
#6301=EDGE_LOOP ( 'NONE', ( #8651, #4322, #9671, #2472 ) ) ;
#6314=AXIS2_PLACEMENT_3D ( 'NONE', #9654, #2830, #5168 ) ;
#6321=DIRECTION ( 'NONE',  ( 0.1666666666666662411, 3.900547397768555245E-29, 0.9860132971832694659 ) ) ;
#6327=DIRECTION ( 'NONE',  ( -1.820952055660014662E-28, -1.000000000000000000, -7.038118388768679669E-30 ) ) ;
#6328=EDGE_LOOP ( 'NONE', ( #1535, #9625, #8660, #3577 ) ) ;
#6341=CARTESIAN_POINT ( 'NONE',  ( 9.860761315262647568E-27, 49.00000000000032685, -25.00000000000000000 ) ) ;
#6343=DIRECTION ( 'NONE',  ( -1.735493991486225972E-29, 6.508102468073347395E-30, 1.000000000000000000 ) ) ;
#6349=LINE ( 'NONE', #9366, #2346 ) ;
#6351=DIRECTION ( 'NONE',  ( -1.735493991486225972E-29, 6.508102468073347395E-30, 1.000000000000000000 ) ) ;
#6357=ADVANCED_FACE ( 'NONE', ( #30 ), #3827, .F. ) ;
#6359=LINE ( 'NONE', #2603, #892 ) ;
#6360=DIRECTION ( 'NONE',  ( 1.735493991486226532E-29, 0.000000000000000000, -1.000000000000000000 ) ) ;
#6365=ORIENTED_EDGE ( 'NONE', *, *, #5284, .T. ) ;
#6368=CIRCLE ( 'NONE', #8431, 26.00000000000000355 ) ;
#6372=AXIS2_PLACEMENT_3D ( 'NONE', #5032, #8002, #8146 ) ;
#6374=EDGE_LOOP ( 'NONE', ( #3326, #114, #1620, #364 ) ) ;
#6378=ORIENTED_EDGE ( 'NONE', *, *, #2249, .F. ) ;
#6384=CARTESIAN_POINT ( 'NONE',  ( -8.216777476527294510, 43.00000000000019895, -23.61111111111111427 ) ) ;
#6391=PLANE ( 'NONE',  #1604 ) ;
#6398=VECTOR ( 'NONE', #6710, 1000.000000000000341 ) ;
#6399=DIRECTION ( 'NONE',  ( -0.9860132971832694659, -1.788557213313974350E-28, 0.1666666666666658247 ) ) ;
#6404=EDGE_LOOP ( 'NONE', ( #5331, #7658, #4289, #6513 ) ) ;
#6411=DIRECTION ( 'NONE',  ( -1.820952055660014662E-28, -1.000000000000000000, -7.038118388768679669E-30 ) ) ;
#6416=LINE ( 'NONE', #4760, #5404 ) ;
#6417=PLANE ( 'NONE',  #5767 ) ;
#6423=VERTEX_POINT ( 'NONE', #375 ) ;
#6446=DIRECTION ( 'NONE',  ( 1.735493991486223450E-29, 0.000000000000000000, -1.000000000000000000 ) ) ;
#6450=CARTESIAN_POINT ( 'NONE',  ( -8.545448575588370232, 56.50000000000029843, -24.55555555555557490 ) ) ;
#6455=CARTESIAN_POINT ( 'NONE',  ( 1.193152119146780356E-26, 58.00000000000029132, -37.00000000000000711 ) ) ;
#6464=ADVANCED_FACE ( 'NONE', ( #7024 ), #9412, .F. ) ;
#6484=PLANE ( 'NONE',  #3300 ) ;
#6492=ADVANCED_FACE ( 'NONE', ( #7974 ), #2520, .T. ) ;
#6495=CARTESIAN_POINT ( 'NONE',  ( 1.040310318760209318E-26, 50.00000000000032685, -37.00000000000000711 ) ) ;
#6498=DIRECTION ( 'NONE',  ( 1.735493991486225972E-29, -6.508102468073347395E-30, -1.000000000000000000 ) ) ;
#6499=FACE_OUTER_BOUND ( 'NONE', #6165, .T. ) ;
#6513=ORIENTED_EDGE ( 'NONE', *, *, #6721, .T. ) ;
#6518=DIRECTION ( 'NONE',  ( 1.735493991486223450E-29, 0.000000000000000000, -1.000000000000000000 ) ) ;
#6520=CARTESIAN_POINT ( 'NONE',  ( 1.555535097482682654E-26, 78.08723716182652197, -25.00000000000000000 ) ) ;
#6521=VERTEX_POINT ( 'NONE', #1939 ) ;
#6528=VECTOR ( 'NONE', #5221, 1000.000000000000000 ) ;
#6539=FACE_OUTER_BOUND ( 'NONE', #5359, .T. ) ;
#6546=ORIENTED_EDGE ( 'NONE', *, *, #1780, .F. ) ;
#6552=CARTESIAN_POINT ( 'NONE',  ( -8.216777476527294510, 56.50000000000029843, -23.61111111111111427 ) ) ;
#6566=CARTESIAN_POINT ( 'NONE',  ( 9.762153702110021092E-27, 46.00000000000018474, -25.00000000000000000 ) ) ;
#6572=ORIENTED_EDGE ( 'NONE', *, *, #8555, .T. ) ;
#6575=DIRECTION ( 'NONE',  ( 1.820952055660014662E-28, 1.000000000000000000, 7.038118388768679669E-30 ) ) ;
#6579=CARTESIAN_POINT ( 'NONE',  ( -8.216777476527294510, 53.50000000000031264, -23.61111111111107519 ) ) ;
#6585=DIRECTION ( 'NONE',  ( 0.3286710990610922090, 6.289316826390952918E-29, 0.9444444444444435316 ) ) ;
#6591=CARTESIAN_POINT ( 'NONE',  ( 8.776077570583756335E-27, 49.00000000000032685, -24.09806918451531033 ) ) ;
#6594=LINE ( 'NONE', #9522, #7760 ) ;
#6597=ADVANCED_FACE ( 'NONE', ( #7426 ), #2167, .F. ) ;
#6606=VECTOR ( 'NONE', #3364, 1000.000000000000341 ) ;
#6613=VERTEX_POINT ( 'NONE', #2078 ) ;
#6614=LINE ( 'NONE', #8897, #7178 ) ;
#6620=VERTEX_POINT ( 'NONE', #2919 ) ;
#6623=ORIENTED_EDGE ( 'NONE', *, *, #5990, .F. ) ;
#6628=CARTESIAN_POINT ( 'NONE',  ( 1.555535097482682654E-26, 78.08723716182652197, -25.00000000000000000 ) ) ;
#6629=DIRECTION ( 'NONE',  ( 1.735493991486225972E-29, -6.508102468073347395E-30, -1.000000000000000000 ) ) ;
#6634=DIRECTION ( 'NONE',  ( -0.3286710990610922090, -6.289316826390952918E-29, -0.9444444444444435316 ) ) ;
#6635=DIRECTION ( 'NONE',  ( -1.820952055660014662E-28, -1.000000000000000000, -7.038118388768679669E-30 ) ) ;
#6638=CARTESIAN_POINT ( 'NONE',  ( 9.269115636346888714E-27, 44.00000000000019895, -37.00000000000000711 ) ) ;
#6643=CARTESIAN_POINT ( 'NONE',  ( 1.555535097482682654E-26, 78.08723716182652197, -25.00000000000000000 ) ) ;
#6648=VECTOR ( 'NONE', #2198, 1000.000000000000000 ) ;
#6649=EDGE_CURVE ( 'NONE', #8408, #1910, #8768, .T. ) ;
#6651=CARTESIAN_POINT ( 'NONE',  ( 9.469456053449529731E-27, 52.00000000000031974, 3.146969529128743384E-28 ) ) ;
#6660=VERTEX_POINT ( 'NONE', #713 ) ;
#6677=AXIS2_PLACEMENT_3D ( 'NONE', #4288, #7993, #1275 ) ;
#6678=CARTESIAN_POINT ( 'NONE',  ( 8.677469957431129860E-27, 40.00000000000014921, -25.00000000000000000 ) ) ;
#6683=CARTESIAN_POINT ( 'NONE',  ( 1.555535097482682654E-26, 78.08723716182652197, -25.00000000000000000 ) ) ;
#6689=AXIS2_PLACEMENT_3D ( 'NONE', #6970, #5510, #6827 ) ;
#6698=LINE ( 'NONE', #9727, #4160 ) ;
#6701=LINE ( 'NONE', #8987, #6648 ) ;
#6709=VERTEX_POINT ( 'NONE', #4561 ) ;
#6710=DIRECTION ( 'NONE',  ( -0.9860132971832693549, -1.788557213313974126E-28, 0.1666666666666657970 ) ) ;
#6713=DIRECTION ( 'NONE',  ( -1.820952055660014662E-28, -1.000000000000000000, -7.038118388768679669E-30 ) ) ;
#6715=DIRECTION ( 'NONE',  ( 1.820952055660014662E-28, 1.000000000000000000, -6.508102468073347395E-30 ) ) ;
#6716=ORIENTED_EDGE ( 'NONE', *, *, #5719, .F. ) ;
#6719=DIRECTION ( 'NONE',  ( -1.820952055660014662E-28, -1.000000000000000000, -7.038118388768679669E-30 ) ) ;
#6721=EDGE_CURVE ( 'NONE', #5636, #7720, #5352, .T. ) ;
#6722=ADVANCED_FACE ( 'NONE', ( #2415 ), #3062, .F. ) ;
#6723=AXIS2_PLACEMENT_3D ( 'NONE', #6591, #5856, #1411 ) ;
#6724=ORIENTED_EDGE ( 'NONE', *, *, #8665, .F. ) ;
#6732=ORIENTED_EDGE ( 'NONE', *, *, #2828, .T. ) ;
#6737=CARTESIAN_POINT ( 'NONE',  ( 1.057802637207955558E-26, 58.00000000000029132, 3.077636051130802893E-28 ) ) ;
#6740=FACE_OUTER_BOUND ( 'NONE', #3370, .T. ) ;
#6746=CARTESIAN_POINT ( 'NONE',  ( 1.148778693228098442E-26, 59.00000000000029843, -24.09806918451521440 ) ) ;
#6760=CARTESIAN_POINT ( 'NONE',  ( 1.084683744678891232E-26, 58.00000000000029132, -24.09806918451521440 ) ) ;
#6769=ORIENTED_EDGE ( 'NONE', *, *, #1848, .T. ) ;
#6775=DIRECTION ( 'NONE',  ( -1.820952055660014662E-28, -1.000000000000000000, -7.038118388768679669E-30 ) ) ;
#6781=( GEOMETRIC_REPRESENTATION_CONTEXT ( 3 ) GLOBAL_UNCERTAINTY_ASSIGNED_CONTEXT ( ( #2277 ) ) GLOBAL_UNIT_ASSIGNED_CONTEXT ( ( #147, #4728, #9226 ) ) REPRESENTATION_CONTEXT ( 'NONE', 'WORKASPACE' ) );
#6783=DIRECTION ( 'NONE',  ( 0.3286710990610922090, 6.289316826390952918E-29, 0.9444444444444435316 ) ) ;
#6787=CARTESIAN_POINT ( 'NONE',  ( 9.762153702110021092E-27, 42.50000000000020606, -37.00000000000000711 ) ) ;
#6789=DIRECTION ( 'NONE',  ( 1.735493991486227934E-29, 0.000000000000000000, -1.000000000000000000 ) ) ;
#6793=VECTOR ( 'NONE', #3181, 1000.000000000000000 ) ;
#6809=CARTESIAN_POINT ( 'NONE',  ( 8.831777707322487581E-27, 48.50000000000033396, 2.950524674801245327E-28 ) ) ;
#6813=CYLINDRICAL_SURFACE ( 'NONE', #9719, 26.00000000000004974 ) ;
#6825=CARTESIAN_POINT ( 'NONE',  ( 0.000000000000000000, 0.000000000000000000, 0.000000000000000000 ) ) ;
#6827=DIRECTION ( 'NONE',  ( -0.9860132971832694659, -1.788557213313974350E-28, 0.1666666666666658247 ) ) ;
#6836=PLANE ( 'NONE',  #5631 ) ;
#6847=CARTESIAN_POINT ( 'NONE',  ( -8.216777476527294510, 45.50000000000019185, -23.61111111111111427 ) ) ;
#6860=EDGE_LOOP ( 'NONE', ( #100, #9164, #3452, #6159 ) ) ;
#6861=CARTESIAN_POINT ( 'NONE',  ( 1.148778693228098442E-26, 55.00000000000030553, -25.00000000000000000 ) ) ;
#6864=DIRECTION ( 'NONE',  ( -0.9860132971832693549, -1.787355433028676715E-28, 0.1666666666666661856 ) ) ;
#6873=CARTESIAN_POINT ( 'NONE',  ( 1.193152119146780356E-26, 56.00000000000030553, -37.00000000000000711 ) ) ;
#6874=ORIENTED_EDGE ( 'NONE', *, *, #4492, .F. ) ;
#6875=ORIENTED_EDGE ( 'NONE', *, *, #8665, .T. ) ;
#6891=DIRECTION ( 'NONE',  ( 1.820952055660014662E-28, 1.000000000000000000, -6.508102468073347395E-30 ) ) ;
#6892=VERTEX_POINT ( 'NONE', #2614 ) ;
#6900=EDGE_CURVE ( 'NONE', #3082, #8311, #6416, .T. ) ;
#6910=DIRECTION ( 'NONE',  ( -1.735493991486225972E-29, 6.508102468073347395E-30, 1.000000000000000000 ) ) ;
#6926=ORIENTED_EDGE ( 'NONE', *, *, #574, .T. ) ;
#6929=EDGE_LOOP ( 'NONE', ( #3924, #8406, #6020, #6926, #9729, #6078, #1829, #8298, #1581, #6193, #798, #3866, #706, #3005, #408, #9546, #6875, #4170, #7531, #3042, #2385, #8461, #5099, #7108, #8764, #2218, #5582, #7382, #4363, #7277, #729, #4660, #7369, #698, #3880, #6086, #6572, #111, #4963, #501, #369, #321, #7303, #9063, #5371, #5547, #6983, #4980, #1844, #4742, #781, #1895 ) ) ;
#6948=EDGE_CURVE ( 'NONE', #9587, #987, #4806, .T. ) ;
#6949=CARTESIAN_POINT ( 'NONE',  ( 1.021055725781022764E-26, 56.00000000000030553, 3.016006292910411346E-28 ) ) ;
#6951=EDGE_CURVE ( 'NONE', #49, #8403, #7763, .T. ) ;
#6966=EDGE_LOOP ( 'NONE', ( #3971, #6365, #3772, #8571 ) ) ;
#6970=CARTESIAN_POINT ( 'NONE',  ( 1.555535097482682654E-26, 78.08723716182652197, -25.00000000000000000 ) ) ;
#6972=VECTOR ( 'NONE', #6719, 1000.000000000000000 ) ;
#6975=VECTOR ( 'NONE', #4994, 1000.000000000000000 ) ;
#6976=VERTEX_POINT ( 'NONE', #9342 ) ;
#6983=ORIENTED_EDGE ( 'NONE', *, *, #9566, .T. ) ;
#6984=DIRECTION ( 'NONE',  ( -1.820952055660014662E-28, -1.000000000000000000, -7.038118388768679669E-30 ) ) ;
#6987=VERTEX_POINT ( 'NONE', #4452 ) ;
#6996=VERTEX_POINT ( 'NONE', #3503 ) ;
#6998=LINE ( 'NONE', #265, #7352 ) ;
#7000=EDGE_LOOP ( 'NONE', ( #5820, #1819, #1800, #7868 ) ) ;
#7011=VERTEX_POINT ( 'NONE', #6566 ) ;
#7013=AXIS2_PLACEMENT_3D ( 'NONE', #1197, #6321, #7814 ) ;
#7022=EDGE_CURVE ( 'NONE', #517, #185, #8050, .T. ) ;
#7023=EDGE_CURVE ( 'NONE', #9740, #6423, #9630, .T. ) ;
#7024=FACE_OUTER_BOUND ( 'NONE', #7970, .T. ) ;
#7030=VERTEX_POINT ( 'NONE', #3557 ) ;
#7031=FACE_OUTER_BOUND ( 'NONE', #7315, .T. ) ;
#7039=FACE_OUTER_BOUND ( 'NONE', #6243, .T. ) ;
#7048=LINE ( 'NONE', #1827, #8933 ) ;
#7049=EDGE_CURVE ( 'NONE', #3249, #7994, #9190, .T. ) ;
#7058=CARTESIAN_POINT ( 'NONE',  ( -8.545448575588396878, -1.822314913379202564E-27, -24.55555555555564951 ) ) ;
#7071=VERTEX_POINT ( 'NONE', #2899 ) ;
#7085=VECTOR ( 'NONE', #7497, 1000.000000000000000 ) ;
#7091=CARTESIAN_POINT ( 'NONE',  ( 7.285056225244056734E-27, 40.00000000000013500, 2.827265158360462232E-28 ) ) ;
#7093=EDGE_CURVE ( 'NONE', #3873, #4022, #5143, .T. ) ;
#7094=EDGE_LOOP ( 'NONE', ( #5468, #3331, #6732, #8216 ) ) ;
#7108=ORIENTED_EDGE ( 'NONE', *, *, #8910, .T. ) ;
#7113=VERTEX_POINT ( 'NONE', #5731 ) ;
#7116=ORIENTED_EDGE ( 'NONE', *, *, #7201, .F. ) ;
#7122=DIRECTION ( 'NONE',  ( 0.1178511301977574338, 0.7071067811865470176, 0.6972166887783970424 ) ) ;
#7125=ORIENTED_EDGE ( 'NONE', *, *, #3169, .T. ) ;
#7126=ORIENTED_EDGE ( 'NONE', *, *, #5350, .T. ) ;
#7127=CARTESIAN_POINT ( 'NONE',  ( 1.555535097482682654E-26, 78.08723716182652197, -25.00000000000000000 ) ) ;
#7143=DIRECTION ( 'NONE',  ( -1.820952055660014662E-28, -1.000000000000000000, 6.508102468073347395E-30 ) ) ;
#7146=EDGE_CURVE ( 'NONE', #7876, #6976, #1681, .T. ) ;
#7150=ADVANCED_FACE ( 'NONE', ( #7608 ), #7705, .F. ) ;
#7153=DIRECTION ( 'NONE',  ( -1.820952055660014662E-28, -1.000000000000000000, -7.038118388768679669E-30 ) ) ;
#7155=CARTESIAN_POINT ( 'NONE',  ( 9.219811829770575476E-27, 50.50000000000031974, -26.00000000000008171 ) ) ;
#7170=ORIENTED_EDGE ( 'NONE', *, *, #9460, .F. ) ;
#7178=VECTOR ( 'NONE', #8159, 1000.000000000000000 ) ;
#7185=LINE ( 'NONE', #2827, #4566 ) ;
#7189=DIRECTION ( 'NONE',  ( -1.820952055660014662E-28, -1.000000000000000000, -7.038118388768679669E-30 ) ) ;
#7190=VECTOR ( 'NONE', #6575, 1000.000000000000000 ) ;
#7201=EDGE_CURVE ( 'NONE', #2421, #6620, #8398, .T. ) ;
#7202=AXIS2_PLACEMENT_3D ( 'NONE', #8137, #8182, #1512 ) ;
#7210=ORIENTED_EDGE ( 'NONE', *, *, #5991, .F. ) ;
#7217=DIRECTION ( 'NONE',  ( -0.1666666666666658525, -3.897465909857536228E-29, -0.9860132971832695770 ) ) ;
#7220=CARTESIAN_POINT ( 'NONE',  ( -8.216777476527274970, 47.50000000000033396, -23.61111111111111427 ) ) ;
#7222=ORIENTED_EDGE ( 'NONE', *, *, #3745, .F. ) ;
#7225=EDGE_CURVE ( 'NONE', #3225, #2857, #3752, .T. ) ;
#7237=EDGE_CURVE ( 'NONE', #4569, #5208, #6701, .T. ) ;
#7238=PLANE ( 'NONE',  #5364 ) ;
#7239=ORIENTED_EDGE ( 'NONE', *, *, #2116, .F. ) ;
#7243=FACE_OUTER_BOUND ( 'NONE', #5472, .T. ) ;
#7255=ORIENTED_EDGE ( 'NONE', *, *, #7022, .F. ) ;
#7267=ORIENTED_EDGE ( 'NONE', *, *, #463, .T. ) ;
#7270=EDGE_CURVE ( 'NONE', #7461, #3950, #5707, .T. ) ;
#7272=EDGE_CURVE ( 'NONE', #3069, #5730, #3046, .T. ) ;
#7277=ORIENTED_EDGE ( 'NONE', *, *, #2248, .T. ) ;
#7279=DIRECTION ( 'NONE',  ( -1.820952055660014662E-28, -1.000000000000000000, -7.038118388768679669E-30 ) ) ;
#7284=AXIS2_PLACEMENT_3D ( 'NONE', #733, #4435, #883 ) ;
#7285=DIRECTION ( 'NONE',  ( -1.735493991486225972E-29, 6.508102468073347395E-30, 1.000000000000000000 ) ) ;
#7290=DIRECTION ( 'NONE',  ( 1.735493991486228214E-29, 0.000000000000000000, -1.000000000000000000 ) ) ;
#7292=ORIENTED_EDGE ( 'NONE', *, *, #3562, .F. ) ;
#7293=DIRECTION ( 'NONE',  ( 0.3286710990610922090, 6.289316826390952918E-29, 0.9444444444444435316 ) ) ;
#7294=CARTESIAN_POINT ( 'NONE',  ( 9.219811829770575476E-27, 50.50000000000031974, -24.09806918451529612 ) ) ;
#7296=VECTOR ( 'NONE', #5885, 1000.000000000000000 ) ;
#7301=ORIENTED_EDGE ( 'NONE', *, *, #2487, .F. ) ;
#7303=ORIENTED_EDGE ( 'NONE', *, *, #3729, .T. ) ;
#7307=CARTESIAN_POINT ( 'NONE',  ( 1.203012880462043003E-26, 59.00000000000029843, -25.00000000000000000 ) ) ;
#7309=CARTESIAN_POINT ( 'NONE',  ( 1.148778693228098442E-26, 51.50000000000032685, -37.00000000000000711 ) ) ;
#7311=ORIENTED_EDGE ( 'NONE', *, *, #9031, .F. ) ;
#7315=EDGE_LOOP ( 'NONE', ( #5076, #8449, #3318, #6724 ) ) ;
#7322=DIRECTION ( 'NONE',  ( -1.820952055660014662E-28, -1.000000000000000000, -7.038118388768679669E-30 ) ) ;
#7326=DIRECTION ( 'NONE',  ( 1.735493991486225972E-29, -6.508102468073347395E-30, -1.000000000000000000 ) ) ;
#7331=CIRCLE ( 'NONE', #1033, 26.00000000000009592 ) ;
#7333=PLANE ( 'NONE',  #2657 ) ;
#7345=PLANE ( 'NONE',  #6723 ) ;
#7349=ORIENTED_EDGE ( 'NONE', *, *, #4474, .F. ) ;
#7352=VECTOR ( 'NONE', #8647, 1000.000000000000000 ) ;
#7369=ORIENTED_EDGE ( 'NONE', *, *, #2956, .T. ) ;
#7377=DIRECTION ( 'NONE',  ( -1.735493991486225972E-29, 6.508102468073347395E-30, 1.000000000000000000 ) ) ;
#7381=VERTEX_POINT ( 'NONE', #302 ) ;
#7382=ORIENTED_EDGE ( 'NONE', *, *, #8849, .T. ) ;
#7388=DIRECTION ( 'NONE',  ( -1.735493991486225972E-29, 6.508102468073347395E-30, 1.000000000000000000 ) ) ;
#7390=EDGE_CURVE ( 'NONE', #1910, #478, #3198, .T. ) ;
#7395=LINE ( 'NONE', #2233, #3399 ) ;
#7396=CARTESIAN_POINT ( 'NONE',  ( -8.216777476527294510, 44.00000000000019895, -23.61111111111111427 ) ) ;
#7397=DIRECTION ( 'NONE',  ( -1.820952055660014662E-28, -1.000000000000000000, 6.508102468073347395E-30 ) ) ;
#7412=VECTOR ( 'NONE', #4034, 1000.000000000000000 ) ;
#7414=DIRECTION ( 'NONE',  ( 1.735493991486225972E-29, -6.508102468073347395E-30, -1.000000000000000000 ) ) ;
#7417=ORIENTED_EDGE ( 'NONE', *, *, #2687, .T. ) ;
#7424=ORIENTED_EDGE ( 'NONE', *, *, #710, .T. ) ;
#7426=FACE_OUTER_BOUND ( 'NONE', #3792, .T. ) ;
#7435=AXIS2_PLACEMENT_3D ( 'NONE', #2682, #3336, #6343 ) ;
#7437=CARTESIAN_POINT ( 'NONE',  ( 1.094544505994153880E-26, 56.50000000000029843, -25.00000000000000000 ) ) ;
#7442=CARTESIAN_POINT ( 'NONE',  ( -8.545448575588393325, 51.50000000000032685, -24.55555555555559621 ) ) ;
#7443=AXIS2_PLACEMENT_3D ( 'NONE', #3490, #3542, #6498 ) ;
#7444=CARTESIAN_POINT ( 'NONE',  ( 8.677469957431129860E-27, 43.00000000000019895, -26.00000000000015987 ) ) ;
#7445=DIRECTION ( 'NONE',  ( -0.9860132971832694659, -1.788557213313974350E-28, 0.1666666666666658247 ) ) ;
#7455=ORIENTED_EDGE ( 'NONE', *, *, #4474, .T. ) ;
#7457=EDGE_CURVE ( 'NONE', #5928, #6521, #9016, .T. ) ;
#7461=VERTEX_POINT ( 'NONE', #3493 ) ;
#7472=ORIENTED_EDGE ( 'NONE', *, *, #8007, .F. ) ;
#7479=LINE ( 'NONE', #5942, #1729 ) ;
#7480=LINE ( 'NONE', #4384, #3795 ) ;
#7481=DIRECTION ( 'NONE',  ( -1.820952055660014662E-28, -1.000000000000000000, -7.038118388768679669E-30 ) ) ;
#7482=AXIS2_PLACEMENT_3D ( 'NONE', #6825, #4529, #5410 ) ;
#7491=DIRECTION ( 'NONE',  ( 1.735493991486228494E-29, 0.000000000000000000, -1.000000000000000000 ) ) ;
#7497=DIRECTION ( 'NONE',  ( 1.820952055660014662E-28, 1.000000000000000000, 7.038118388768679669E-30 ) ) ;
#7500=DIRECTION ( 'NONE',  ( -1.820952055660014662E-28, -1.000000000000000000, -7.038118388768679669E-30 ) ) ;
#7501=VECTOR ( 'NONE', #8972, 1000.000000000000341 ) ;
#7508=EDGE_CURVE ( 'NONE', #1296, #1637, #4988, .T. ) ;
#7514=EDGE_CURVE ( 'NONE', #3045, #6709, #3547, .T. ) ;
#7518=EDGE_CURVE ( 'NONE', #8065, #3624, #8000, .T. ) ;
#7519=VECTOR ( 'NONE', #3543, 1000.000000000000000 ) ;
#7520=CARTESIAN_POINT ( 'NONE',  ( 8.283039504820623957E-27, 47.00000000000034106, -26.00000000000012790 ) ) ;
#7524=VERTEX_POINT ( 'NONE', #8789 ) ;
#7529=EDGE_CURVE ( 'NONE', #2848, #4270, #8093, .T. ) ;
#7530=VECTOR ( 'NONE', #7635, 1000.000000000000114 ) ;
#7531=ORIENTED_EDGE ( 'NONE', *, *, #4563, .T. ) ;
#7536=ORIENTED_EDGE ( 'NONE', *, *, #226, .F. ) ;
#7537=PLANE ( 'NONE',  #4414 ) ;
#7542=VERTEX_POINT ( 'NONE', #5817 ) ;
#7550=CARTESIAN_POINT ( 'NONE',  ( -8.545448575588403983, -1.753944400353455691E-27, -24.55555555555566727 ) ) ;
#7556=CARTESIAN_POINT ( 'NONE',  ( 0.000000000000000000, 0.000000000000000000, 0.000000000000000000 ) ) ;
#7576=VECTOR ( 'NONE', #7839, 1000.000000000000000 ) ;
#7587=ORIENTED_EDGE ( 'NONE', *, *, #6251, .F. ) ;
#7601=ORIENTED_EDGE ( 'NONE', *, *, #3284, .F. ) ;
#7608=FACE_OUTER_BOUND ( 'NONE', #3187, .T. ) ;
#7609=CARTESIAN_POINT ( 'NONE',  ( 9.762153702110021092E-27, 46.00000000000018474, -37.00000000000000711 ) ) ;
#7610=VERTEX_POINT ( 'NONE', #2476 ) ;
#7613=ORIENTED_EDGE ( 'NONE', *, *, #7146, .F. ) ;
#7614=FACE_OUTER_BOUND ( 'NONE', #8903, .T. ) ;
#7615=CARTESIAN_POINT ( 'NONE',  ( -8.216777476527294510, 46.00000000000018474, -23.61111111111111427 ) ) ;
#7618=ORIENTED_EDGE ( 'NONE', *, *, #1978, .T. ) ;
#7622=LINE ( 'NONE', #2416, #2238 ) ;
#7634=EDGE_LOOP ( 'NONE', ( #3079, #9702, #9472, #8071 ) ) ;
#7635=DIRECTION ( 'NONE',  ( -1.301620493614667237E-28, -0.7021094974994117610, 0.7120689949163097054 ) ) ;
#7658=ORIENTED_EDGE ( 'NONE', *, *, #8073, .T. ) ;
#7660=CIRCLE ( 'NONE', #9408, 26.00000000000003197 ) ;
#7661=CARTESIAN_POINT ( 'NONE',  ( -8.545448575588380891, 53.50000000000031264, -24.55555555555556779 ) ) ;
#7667=LINE ( 'NONE', #6861, #6398 ) ;
#7668=CARTESIAN_POINT ( 'NONE',  ( 8.934430193578387011E-27, 49.00000000000032685, 3.243266026348105177E-28 ) ) ;
#7677=VECTOR ( 'NONE', #8585, 1000.000000000000000 ) ;
#7678=ORIENTED_EDGE ( 'NONE', *, *, #7049, .F. ) ;
#7683=DIRECTION ( 'NONE',  ( 1.735493991486225972E-29, -6.508102468073347395E-30, -1.000000000000000000 ) ) ;
#7690=CARTESIAN_POINT ( 'NONE',  ( 1.093393990668256298E-26, 60.00000000000029843, 3.177784408238939158E-28 ) ) ;
#7696=LINE ( 'NONE', #7789, #3228 ) ;
#7705=PLANE ( 'NONE',  #358 ) ;
#7717=CARTESIAN_POINT ( 'NONE',  ( 1.084683744678891232E-26, 50.50000000000031974, -37.00000000000000711 ) ) ;
#7720=VERTEX_POINT ( 'NONE', #284 ) ;
#7722=AXIS2_PLACEMENT_3D ( 'NONE', #6949, #3354, #6360 ) ;
#7750=ORIENTED_EDGE ( 'NONE', *, *, #8852, .T. ) ;
#7759=CARTESIAN_POINT ( 'NONE',  ( 1.040310318760209318E-26, 50.00000000000032685, -25.00000000000000000 ) ) ;
#7760=VECTOR ( 'NONE', #7293, 1000.000000000000000 ) ;
#7763=LINE ( 'NONE', #2563, #2068 ) ;
#7772=ORIENTED_EDGE ( 'NONE', *, *, #3870, .T. ) ;
#7782=CARTESIAN_POINT ( 'NONE',  ( 1.084683744678891232E-26, 53.00000000000031974, -25.00000000000000000 ) ) ;
#7784=CARTESIAN_POINT ( 'NONE',  ( -8.216777476527294510, 59.00000000000029843, -23.61111111111111427 ) ) ;
#7786=CARTESIAN_POINT ( 'NONE',  ( -8.545448575588393325, 45.50000000000019185, -24.55555555555569569 ) ) ;
#7789=CARTESIAN_POINT ( 'NONE',  ( 1.148778693228098442E-26, 57.50000000000029843, -37.00000000000000711 ) ) ;
#7790=EDGE_CURVE ( 'NONE', #478, #6987, #9499, .T. ) ;
#7794=VERTEX_POINT ( 'NONE', #5744 ) ;
#7805=VECTOR ( 'NONE', #1871, 1000.000000000000000 ) ;
#7814=DIRECTION ( 'NONE',  ( 0.9860132971832693549, 1.788449361237088441E-28, -0.1666666666666662133 ) ) ;
#7815=AXIS2_PLACEMENT_3D ( 'NONE', #777, #9663, #628 ) ;
#7820=EDGE_LOOP ( 'NONE', ( #2514, #2335, #7587, #481 ) ) ;
#7823=VECTOR ( 'NONE', #3101, 1000.000000000000000 ) ;
#7825=CARTESIAN_POINT ( 'NONE',  ( 1.094544505994153880E-26, 60.00000000000029843, -26.01418510567422970 ) ) ;
#7831=EDGE_CURVE ( 'NONE', #6892, #4799, #3325, .T. ) ;
#7835=EDGE_CURVE ( 'NONE', #7876, #1008, #7927, .T. ) ;
#7837=EDGE_CURVE ( 'NONE', #2117, #3682, #9356, .T. ) ;
#7839=DIRECTION ( 'NONE',  ( -0.2340364991664707905, 0.7021094974994116500, -0.6725096063098476851 ) ) ;
#7848=CARTESIAN_POINT ( 'NONE',  ( 8.874685183736382811E-27, 44.50000000000019185, -26.00000000000014566 ) ) ;
#7853=DIRECTION ( 'NONE',  ( 0.3286710990610922090, 6.289316826390952918E-29, 0.9444444444444435316 ) ) ;
#7860=CARTESIAN_POINT ( 'NONE',  ( 5.423418723394456162E-28, -2.066522830327504070E-28, -26.00000000000002132 ) ) ;
#7861=CARTESIAN_POINT ( 'NONE',  ( 1.138917931912835794E-26, 53.50000000000031264, -37.00000000000000711 ) ) ;
#7864=CARTESIAN_POINT ( 'NONE',  ( 1.148778693228098442E-26, 57.50000000000029843, -26.00000000000002132 ) ) ;
#7868=ORIENTED_EDGE ( 'NONE', *, *, #3038, .T. ) ;
#7873=LINE ( 'NONE', #9452, #103 ) ;
#7876=VERTEX_POINT ( 'NONE', #5203 ) ;
#7891=EDGE_CURVE ( 'NONE', #7610, #7994, #5937, .T. ) ;
#7895=ORIENTED_EDGE ( 'NONE', *, *, #1108, .T. ) ;
#7913=DIRECTION ( 'NONE',  ( -0.3286710990610922090, -6.289316826390952918E-29, -0.9444444444444435316 ) ) ;
#7915=EDGE_CURVE ( 'NONE', #3824, #1005, #5251, .T. ) ;
#7922=LINE ( 'NONE', #1207, #3879 ) ;
#7927=LINE ( 'NONE', #4961, #4785 ) ;
#7929=PLANE ( 'NONE',  #1892 ) ;
#7938=AXIS2_PLACEMENT_3D ( 'NONE', #1177, #2096, #6446 ) ;
#7940=EDGE_CURVE ( 'NONE', #185, #3249, #1304, .T. ) ;
#7942=ORIENTED_EDGE ( 'NONE', *, *, #9014, .F. ) ;
#7944=CARTESIAN_POINT ( 'NONE',  ( -8.216777476527294510, 40.00000000000014921, -23.61111111111111427 ) ) ;
#7964=VECTOR ( 'NONE', #1326, 1000.000000000000000 ) ;
#7968=DIRECTION ( 'NONE',  ( -1.820952055660014662E-28, -1.000000000000000000, -7.038118388768679669E-30 ) ) ;
#7970=EDGE_LOOP ( 'NONE', ( #4712, #9149, #7417, #6091 ) ) ;
#7974=FACE_OUTER_BOUND ( 'NONE', #1884, .T. ) ;
#7978=VECTOR ( 'NONE', #4171, 1000.000000000000000 ) ;
#7979=ORIENTED_EDGE ( 'NONE', *, *, #8910, .F. ) ;
#7984=DIRECTION ( 'NONE',  ( 1.820952055660014662E-28, 1.000000000000000000, -6.508102468073347395E-30 ) ) ;
#7988=VECTOR ( 'NONE', #2319, 1000.000000000000000 ) ;
#7989=EDGE_CURVE ( 'NONE', #8408, #6709, #3724, .T. ) ;
#7993=DIRECTION ( 'NONE',  ( -1.820952055660014662E-28, -1.000000000000000000, 6.508102468073347395E-30 ) ) ;
#7994=VERTEX_POINT ( 'NONE', #4376 ) ;
#7997=EDGE_CURVE ( 'NONE', #6613, #5960, #4521, .T. ) ;
#8000=LINE ( 'NONE', #8832, #2545 ) ;
#8002=DIRECTION ( 'NONE',  ( -0.1666666666666658525, -3.897465909857536228E-29, -0.9860132971832695770 ) ) ;
#8003=ORIENTED_EDGE ( 'NONE', *, *, #463, .F. ) ;
#8004=DIRECTION ( 'NONE',  ( 0.3286710990610922090, 6.289316826390952918E-29, 0.9444444444444435316 ) ) ;
#8006=VERTEX_POINT ( 'NONE', #9005 ) ;
#8007=EDGE_CURVE ( 'NONE', #2949, #2537, #5799, .T. ) ;
#8018=ORIENTED_EDGE ( 'NONE', *, *, #8538, .F. ) ;
#8032=CARTESIAN_POINT ( 'NONE',  ( 1.555535097482682654E-26, 78.08723716182652197, -25.00000000000000000 ) ) ;
#8033=EDGE_LOOP ( 'NONE', ( #4309, #6716, #5155, #7979 ) ) ;
#8036=ORIENTED_EDGE ( 'NONE', *, *, #4928, .T. ) ;
#8042=DIRECTION ( 'NONE',  ( 1.820952055660014662E-28, 1.000000000000000000, 7.038118388768679669E-30 ) ) ;
#8050=LINE ( 'NONE', #8099, #3015 ) ;
#8059=CARTESIAN_POINT ( 'NONE',  ( 1.555535097482682654E-26, 78.08723716182652197, -25.00000000000000000 ) ) ;
#8060=EDGE_CURVE ( 'NONE', #3135, #2949, #6172, .T. ) ;
#8064=LINE ( 'NONE', #4084, #4046 ) ;
#8065=VERTEX_POINT ( 'NONE', #5308 ) ;
#8066=DIRECTION ( 'NONE',  ( -1.820952055660014662E-28, -1.000000000000000000, -7.038118388768679669E-30 ) ) ;
#8068=AXIS2_PLACEMENT_3D ( 'NONE', #4135, #2528, #4869 ) ;
#8071=ORIENTED_EDGE ( 'NONE', *, *, #2956, .F. ) ;
#8073=EDGE_CURVE ( 'NONE', #9391, #2731, #7622, .T. ) ;
#8093=LINE ( 'NONE', #3025, #5721 ) ;
#8096=DIRECTION ( 'NONE',  ( -1.735493991486225972E-29, 6.508102468073347395E-30, 1.000000000000000000 ) ) ;
#8098=ORIENTED_EDGE ( 'NONE', *, *, #3777, .F. ) ;
#8099=CARTESIAN_POINT ( 'NONE',  ( 1.097009696322969542E-26, 52.00000000000031974, -25.00000000000000000 ) ) ;
#8104=ORIENTED_EDGE ( 'NONE', *, *, #7529, .F. ) ;
#8111=ORIENTED_EDGE ( 'NONE', *, *, #937, .F. ) ;
#8119=ORIENTED_EDGE ( 'NONE', *, *, #684, .F. ) ;
#8120=CARTESIAN_POINT ( 'NONE',  ( 1.555535097482682654E-26, 78.08723716182652197, -25.00000000000000000 ) ) ;
#8123=CARTESIAN_POINT ( 'NONE',  ( 1.040310318760209318E-26, 49.00000000000032685, -37.00000000000000711 ) ) ;
#8136=ORIENTED_EDGE ( 'NONE', *, *, #2444, .T. ) ;
#8137=CARTESIAN_POINT ( 'NONE',  ( 7.557191387046156742E-27, 41.50000000000020606, 2.842672597915560119E-28 ) ) ;
#8139=DIRECTION ( 'NONE',  ( -0.3286710990610922090, -6.289316826390952918E-29, -0.9444444444444435316 ) ) ;
#8141=LINE ( 'NONE', #5717, #5399 ) ;
#8146=DIRECTION ( 'NONE',  ( -0.9860132971832694659, -1.788557213313974350E-28, 0.1666666666666658247 ) ) ;
#8159=DIRECTION ( 'NONE',  ( 1.820952055660014662E-28, 1.000000000000000000, 7.038118388768679669E-30 ) ) ;
#8166=DIRECTION ( 'NONE',  ( -1.820952055660014662E-28, -1.000000000000000000, -7.038118388768679669E-30 ) ) ;
#8173=DIRECTION ( 'NONE',  ( -0.9860132971832693549, -1.788557213313974126E-28, 0.1666666666666657970 ) ) ;
#8182=DIRECTION ( 'NONE',  ( -1.820952055660014662E-28, -1.000000000000000000, -7.038118388768679669E-30 ) ) ;
#8190=FACE_OUTER_BOUND ( 'NONE', #1253, .T. ) ;
#8195=CARTESIAN_POINT ( 'NONE',  ( -8.216777476527274970, 78.08723716182652197, -23.61111111111111427 ) ) ;
#8203=CARTESIAN_POINT ( 'NONE',  ( 1.045240699417840642E-26, 47.50000000000033396, -37.00000000000000711 ) ) ;
#8214=CARTESIAN_POINT ( 'NONE',  ( 0.000000000000000000, 0.000000000000000000, 0.000000000000000000 ) ) ;
#8215=ADVANCED_FACE ( 'NONE', ( #3419 ), #6417, .F. ) ;
#8216=ORIENTED_EDGE ( 'NONE', *, *, #4693, .T. ) ;
#8217=DIRECTION ( 'NONE',  ( -0.9860132971832694659, -1.788557213313974350E-28, 0.1666666666666658247 ) ) ;
#8224=EDGE_CURVE ( 'NONE', #6996, #8006, #5732, .T. ) ;
#8225=CARTESIAN_POINT ( 'NONE',  ( 1.094544505994153880E-26, 56.50000000000029843, -26.00000000000002132 ) ) ;
#8232=EDGE_CURVE ( 'NONE', #2716, #2421, #3459, .T. ) ;
#8235=ADVANCED_FACE ( 'NONE', ( #4949 ), #8606, .F. ) ;
#8239=CARTESIAN_POINT ( 'NONE',  ( 9.762153702110021092E-27, 45.50000000000019185, -25.00000000000000000 ) ) ;
#8240=DIRECTION ( 'NONE',  ( -1.735493991486225972E-29, 6.508102468073347395E-30, 1.000000000000000000 ) ) ;
#8245=DIRECTION ( 'NONE',  ( -1.735493991486225972E-29, 6.508102468073347395E-30, 1.000000000000000000 ) ) ;
#8254=AXIS2_PLACEMENT_3D ( 'NONE', #5114, #7279, #1359 ) ;
#8259=CARTESIAN_POINT ( 'NONE',  ( 1.555535097482682654E-26, 78.08723716182652197, -25.00000000000000000 ) ) ;
#8262=DIRECTION ( 'NONE',  ( -0.3286710990610922090, -6.289316826390952918E-29, -0.9444444444444435316 ) ) ;
#8268=EDGE_LOOP ( 'NONE', ( #7349, #7536, #3, #2780 ) ) ;
#8270=FACE_OUTER_BOUND ( 'NONE', #65, .T. ) ;
#8276=CIRCLE ( 'NONE', #3065, 26.00000000000008171 ) ;
#8278=LINE ( 'NONE', #9661, #7501 ) ;
#8288=VECTOR ( 'NONE', #5589, 1000.000000000000000 ) ;
#8294=VECTOR ( 'NONE', #8316, 1000.000000000000341 ) ;
#8298=ORIENTED_EDGE ( 'NONE', *, *, #7390, .T. ) ;
#8300=VECTOR ( 'NONE', #2635, 1000.000000000000341 ) ;
#8311=VERTEX_POINT ( 'NONE', #5042 ) ;
#8316=DIRECTION ( 'NONE',  ( 0.9860132971832693549, 1.788557213313974126E-28, -0.1666666666666657970 ) ) ;
#8318=EDGE_LOOP ( 'NONE', ( #159, #195, #2621, #9101 ) ) ;
#8324=CARTESIAN_POINT ( 'NONE',  ( 8.455602827837720289E-27, 41.50000000000020606, -24.09806918451538849 ) ) ;
#8333=LINE ( 'NONE', #5994, #5460 ) ;
#8335=FACE_OUTER_BOUND ( 'NONE', #4943, .T. ) ;
#8337=ORIENTED_EDGE ( 'NONE', *, *, #9278, .F. ) ;
#8341=ORIENTED_EDGE ( 'NONE', *, *, #2249, .T. ) ;
#8346=CIRCLE ( 'NONE', #8254, 26.00000000000014566 ) ;
#8355=ORIENTED_EDGE ( 'NONE', *, *, #1108, .F. ) ;
#8356=LINE ( 'NONE', #4614, #2449 ) ;
#8365=EDGE_CURVE ( 'NONE', #7381, #7113, #5236, .T. ) ;
#8370=ORIENTED_EDGE ( 'NONE', *, *, #4260, .F. ) ;
#8385=LINE ( 'NONE', #5518, #8685 ) ;
#8389=ADVANCED_FACE ( 'NONE', ( #9424 ), #2637, .F. ) ;
#8390=VECTOR ( 'NONE', #154, 1000.000000000000341 ) ;
#8397=VECTOR ( 'NONE', #7913, 1000.000000000000000 ) ;
#8398=LINE ( 'NONE', #3701, #3182 ) ;
#8403=VERTEX_POINT ( 'NONE', #2109 ) ;
#8404=CARTESIAN_POINT ( 'NONE',  ( 1.094544505994153880E-26, 55.00000000000030553, -24.09806918451524638 ) ) ;
#8406=ORIENTED_EDGE ( 'NONE', *, *, #649, .T. ) ;
#8407=CARTESIAN_POINT ( 'NONE',  ( -8.216777476527274970, 49.00000000000032685, -23.61111111111111427 ) ) ;
#8408=VERTEX_POINT ( 'NONE', #3702 ) ;
#8409=CARTESIAN_POINT ( 'NONE',  ( 9.318419442923201951E-27, 47.00000000000034106, -25.00000000000000000 ) ) ;
#8416=ORIENTED_EDGE ( 'NONE', *, *, #1780, .T. ) ;
#8431=AXIS2_PLACEMENT_3D ( 'NONE', #3245, #9281, #545 ) ;
#8436=VECTOR ( 'NONE', #8066, 1000.000000000000000 ) ;
#8438=ORIENTED_EDGE ( 'NONE', *, *, #4743, .T. ) ;
#8449=ORIENTED_EDGE ( 'NONE', *, *, #7915, .F. ) ;
#8461=ORIENTED_EDGE ( 'NONE', *, *, #4068, .T. ) ;
#8462=AXIS2_PLACEMENT_3D ( 'NONE', #2027, #9361, #5613 ) ;
#8471=ORIENTED_EDGE ( 'NONE', *, *, #7457, .F. ) ;
#8478=DIRECTION ( 'NONE',  ( -1.820952055660014662E-28, -1.000000000000000000, -7.038118388768679669E-30 ) ) ;
#8481=LINE ( 'NONE', #7784, #2526 ) ;
#8507=VERTEX_POINT ( 'NONE', #119 ) ;
#8512=EDGE_CURVE ( 'NONE', #269, #7542, #3199, .T. ) ;
#8513=EDGE_LOOP ( 'NONE', ( #8599, #1562, #2700, #3361 ) ) ;
#8516=VECTOR ( 'NONE', #4004, 1000.000000000000000 ) ;
#8525=FACE_OUTER_BOUND ( 'NONE', #1797, .T. ) ;
#8528=DIRECTION ( 'NONE',  ( -0.3286710990610922090, -6.289316826390952918E-29, -0.9444444444444435316 ) ) ;
#8530=AXIS2_PLACEMENT_3D ( 'NONE', #5375, #4087, #2342 ) ;
#8538=EDGE_CURVE ( 'NONE', #6892, #8403, #2915, .T. ) ;
#8543=DIRECTION ( 'NONE',  ( 0.9860132971832693549, 1.788557213313974126E-28, -0.1666666666666657970 ) ) ;
#8551=ORIENTED_EDGE ( 'NONE', *, *, #7022, .T. ) ;
#8553=VECTOR ( 'NONE', #4403, 1000.000000000000341 ) ;
#8555=EDGE_CURVE ( 'NONE', #8403, #7011, #8, .T. ) ;
#8566=VECTOR ( 'NONE', #4821, 1000.000000000000000 ) ;
#8571=ORIENTED_EDGE ( 'NONE', *, *, #9204, .T. ) ;
#8572=LINE ( 'NONE', #1751, #7576 ) ;
#8573=ORIENTED_EDGE ( 'NONE', *, *, #468, .F. ) ;
#8581=AXIS2_PLACEMENT_3D ( 'NONE', #5570, #5430, #4697 ) ;
#8585=DIRECTION ( 'NONE',  ( 1.820952055660014662E-28, 1.000000000000000000, 7.038118388768679669E-30 ) ) ;
#8586=ORIENTED_EDGE ( 'NONE', *, *, #1788, .F. ) ;
#8599=ORIENTED_EDGE ( 'NONE', *, *, #1714, .F. ) ;
#8604=VECTOR ( 'NONE', #3855, 1000.000000000000000 ) ;
#8606=PLANE ( 'NONE',  #7013 ) ;
#8607=VECTOR ( 'NONE', #6327, 1000.000000000000000 ) ;
#8612=ORIENTED_EDGE ( 'NONE', *, *, #748, .F. ) ;
#8615=AXIS2_PLACEMENT_3D ( 'NONE', #6019, #6715, #6910 ) ;
#8616=ORIENTED_EDGE ( 'NONE', *, *, #7237, .F. ) ;
#8619=ORIENTED_EDGE ( 'NONE', *, *, #8232, .F. ) ;
#8629=DIRECTION ( 'NONE',  ( 0.9860132971832693549, 1.788557213313974126E-28, -0.1666666666666657970 ) ) ;
#8630=ORIENTED_EDGE ( 'NONE', *, *, #2451, .T. ) ;
#8636=DIRECTION ( 'NONE',  ( -0.1666666666666658525, -3.897465909857536228E-29, -0.9860132971832695770 ) ) ;
#8638=LINE ( 'NONE', #9322, #3854 ) ;
#8647=DIRECTION ( 'NONE',  ( -0.3286710990610922090, -6.289316826390952918E-29, -0.9444444444444435316 ) ) ;
#8651=ORIENTED_EDGE ( 'NONE', *, *, #1407, .F. ) ;
#8660=ORIENTED_EDGE ( 'NONE', *, *, #2674, .T. ) ;
#8665=EDGE_CURVE ( 'NONE', #5592, #5397, #5632, .T. ) ;
#8667=CARTESIAN_POINT ( 'NONE',  ( -8.545448575588407536, -1.821351948407008946E-27, -24.55555555555568148 ) ) ;
#8670=ORIENTED_EDGE ( 'NONE', *, *, #9582, .T. ) ;
#8673=CYLINDRICAL_SURFACE ( 'NONE', #2846, 26.00000000000011369 ) ;
#8674=CYLINDRICAL_SURFACE ( 'NONE', #8462, 26.00000000000014566 ) ;
#8678=EDGE_CURVE ( 'NONE', #2267, #1008, #6359, .T. ) ;
#8685=VECTOR ( 'NONE', #8528, 1000.000000000000000 ) ;
#8690=PLANE ( 'NONE',  #4368 ) ;
#8691=EDGE_LOOP ( 'NONE', ( #611, #7601, #7455, #8874 ) ) ;
#8702=DIRECTION ( 'NONE',  ( 0.3286710990610922090, 6.289316826390952918E-29, 0.9444444444444435316 ) ) ;
#8711=ORIENTED_EDGE ( 'NONE', *, *, #2116, .T. ) ;
#8717=ORIENTED_EDGE ( 'NONE', *, *, #1000, .F. ) ;
#8759=VECTOR ( 'NONE', #5244, 1000.000000000000114 ) ;
#8764=ORIENTED_EDGE ( 'NONE', *, *, #8060, .T. ) ;
#8768=CIRCLE ( 'NONE', #4505, 26.00000000000002132 ) ;
#8781=DIRECTION ( 'NONE',  ( -1.820952055660014662E-28, -1.000000000000000000, -7.038118388768679669E-30 ) ) ;
#8789=CARTESIAN_POINT ( 'NONE',  ( 1.148778693228098442E-26, 55.00000000000030553, -25.00000000000000000 ) ) ;
#8792=PLANE ( 'NONE',  #6372 ) ;
#8803=ORIENTED_EDGE ( 'NONE', *, *, #2623, .F. ) ;
#8804=LINE ( 'NONE', #8203, #4974 ) ;
#8812=CARTESIAN_POINT ( 'NONE',  ( -8.545448575588382667, 54.50000000000031264, -24.55555555555560687 ) ) ;
#8819=EDGE_CURVE ( 'NONE', #1081, #6613, #4136, .T. ) ;
#8822=FACE_OUTER_BOUND ( 'NONE', #4075, .T. ) ;
#8823=ORIENTED_EDGE ( 'NONE', *, *, #7831, .T. ) ;
#8832=CARTESIAN_POINT ( 'NONE',  ( 1.555535097482682654E-26, 78.08723716182652197, -25.00000000000000000 ) ) ;
#8849=EDGE_CURVE ( 'NONE', #2192, #1495, #1802, .T. ) ;
#8851=DIRECTION ( 'NONE',  ( -1.820952055660014662E-28, -1.000000000000000000, -7.038118388768679669E-30 ) ) ;
#8852=EDGE_CURVE ( 'NONE', #5208, #1486, #9640, .T. ) ;
#8853=VERTEX_POINT ( 'NONE', #4830 ) ;
#8871=PRODUCT_DEFINITION ( 'UNKNOWN', '', #2847, #25 ) ;
#8874=ORIENTED_EDGE ( 'NONE', *, *, #1487, .F. ) ;
#8883=CARTESIAN_POINT ( 'NONE',  ( -8.545448575588412865, -1.753174028375700797E-27, -24.55555555555569569 ) ) ;
#8884=CARTESIAN_POINT ( 'NONE',  ( 9.318419442923201951E-27, 44.00000000000019895, -25.00000000000000000 ) ) ;
#8897=CARTESIAN_POINT ( 'NONE',  ( -8.545448575588372009, -1.756640702275597822E-27, -24.55555555555557845 ) ) ;
#8903=EDGE_LOOP ( 'NONE', ( #2893, #1308, #5277, #8337 ) ) ;
#8906=DIRECTION ( 'NONE',  ( -0.3286710990610922090, -6.289316826390952918E-29, -0.9444444444444435316 ) ) ;
#8910=EDGE_CURVE ( 'NONE', #7071, #3135, #8064, .T. ) ;
#8912=ADVANCED_FACE ( 'NONE', ( #1346 ), #8674, .F. ) ;
#8921=VECTOR ( 'NONE', #1291, 1000.000000000000000 ) ;
#8925=LINE ( 'NONE', #6678, #2356 ) ;
#8932=CARTESIAN_POINT ( 'NONE',  ( -8.216777476527294510, 55.00000000000030553, -23.61111111111111427 ) ) ;
#8933=VECTOR ( 'NONE', #7153, 1000.000000000000000 ) ;
#8940=ORIENTED_EDGE ( 'NONE', *, *, #890, .T. ) ;
#8945=DIRECTION ( 'NONE',  ( -1.820952055660014662E-28, -1.000000000000000000, -7.038118388768679669E-30 ) ) ;
#8949=ORIENTED_EDGE ( 'NONE', *, *, #5284, .F. ) ;
#8958=CARTESIAN_POINT ( 'NONE',  ( -8.216777476527294510, 52.00000000000031974, -23.61111111111111427 ) ) ;
#8963=EDGE_LOOP ( 'NONE', ( #2559, #7942, #9451, #8111 ) ) ;
#8969=ADVANCED_FACE ( 'NONE', ( #5931 ), #6813, .F. ) ;
#8972=DIRECTION ( 'NONE',  ( 0.9860132971832693549, 1.788557213313974126E-28, -0.1666666666666657970 ) ) ;
#8975=EDGE_CURVE ( 'NONE', #5960, #9622, #3716, .T. ) ;
#8980=DIRECTION ( 'NONE',  ( -0.1666666666666658525, -3.897465909857536228E-29, -0.9860132971832695770 ) ) ;
#8987=CARTESIAN_POINT ( 'NONE',  ( -8.216777476527294510, 41.50000000000020606, -23.61111111111111427 ) ) ;
#8990=ORIENTED_EDGE ( 'NONE', *, *, #8512, .T. ) ;
#8996=DIRECTION ( 'NONE',  ( 0.9860132971832693549, 1.788557213313974126E-28, -0.1666666666666657970 ) ) ;
#8998=DIRECTION ( 'NONE',  ( -1.820952055660014662E-28, -1.000000000000000000, -7.038118388768679669E-30 ) ) ;
#9001=AXIS2_PLACEMENT_3D ( 'NONE', #2976, #5850, #6629 ) ;
#9005=CARTESIAN_POINT ( 'NONE',  ( 9.811457508686334330E-27, 54.50000000000031264, -26.00000000000004974 ) ) ;
#9013=PLANE ( 'NONE',  #2684 ) ;
#9014=EDGE_CURVE ( 'NONE', #6613, #2714, #3864, .T. ) ;
#9016=LINE ( 'NONE', #1182, #3826 ) ;
#9017=ADVANCED_FACE ( 'NONE', ( #3919 ), #5348, .F. ) ;
#9024=CARTESIAN_POINT ( 'NONE',  ( -8.216777476527274970, 78.08723716182652197, -23.61111111111111427 ) ) ;
#9027=PLANE ( 'NONE',  #8530 ) ;
#9031=EDGE_CURVE ( 'NONE', #6521, #667, #8356, .T. ) ;
#9034=ORIENTED_EDGE ( 'NONE', *, *, #9573, .F. ) ;
#9036=ORIENTED_EDGE ( 'NONE', *, *, #5991, .T. ) ;
#9042=DIRECTION ( 'NONE',  ( 0.9860132971832693549, 1.788557213313974126E-28, -0.1666666666666657970 ) ) ;
#9043=DIRECTION ( 'NONE',  ( 1.735493991486225692E-29, 0.000000000000000000, -1.000000000000000000 ) ) ;
#9053=DIRECTION ( 'NONE',  ( -1.820952055660014662E-28, -1.000000000000000000, -7.038118388768679669E-30 ) ) ;
#9058=AXIS2_PLACEMENT_3D ( 'NONE', #7556, #7500, #5956 ) ;
#9063=ORIENTED_EDGE ( 'NONE', *, *, #7270, .T. ) ;
#9069=DIRECTION ( 'NONE',  ( -1.735493991486225972E-29, 6.508102468073347395E-30, 1.000000000000000000 ) ) ;
#9073=VECTOR ( 'NONE', #4267, 1000.000000000000000 ) ;
#9077=CARTESIAN_POINT ( 'NONE',  ( -8.545448575588377338, 49.00000000000032685, -24.55555555555561043 ) ) ;
#9086=DIRECTION ( 'NONE',  ( 1.820952055660014662E-28, 1.000000000000000000, -6.508102468073347395E-30 ) ) ;
#9092=VERTEX_POINT ( 'NONE', #5199 ) ;
#9099=VERTEX_POINT ( 'NONE', #7759 ) ;
#9101=ORIENTED_EDGE ( 'NONE', *, *, #8849, .F. ) ;
#9111=DIRECTION ( 'NONE',  ( -1.820952055660014662E-28, -1.000000000000000000, -7.038118388768679669E-30 ) ) ;
#9115=VERTEX_POINT ( 'NONE', #2505 ) ;
#9126=VERTEX_POINT ( 'NONE', #309 ) ;
#9131=CYLINDRICAL_SURFACE ( 'NONE', #5987, 26.00000000000012790 ) ;
#9132=ORIENTED_EDGE ( 'NONE', *, *, #9566, .F. ) ;
#9141=DIRECTION ( 'NONE',  ( 1.820952055660014662E-28, 1.000000000000000000, -6.508102468073347395E-30 ) ) ;
#9149=ORIENTED_EDGE ( 'NONE', *, *, #3870, .F. ) ;
#9151=ORIENTED_EDGE ( 'NONE', *, *, #2646, .F. ) ;
#9164=ORIENTED_EDGE ( 'NONE', *, *, #7831, .F. ) ;
#9176=CARTESIAN_POINT ( 'NONE',  ( -8.545448575588382667, -1.755677737303404204E-27, -24.55555555555560687 ) ) ;
#9178=DIRECTION ( 'NONE',  ( -0.9860132971832694659, -1.788557213313974350E-28, 0.1666666666666658247 ) ) ;
#9181=ORIENTED_EDGE ( 'NONE', *, *, #553, .T. ) ;
#9182=DIRECTION ( 'NONE',  ( -0.9860132971832694659, -1.788557213313974350E-28, 0.1666666666666658247 ) ) ;
#9185=CARTESIAN_POINT ( 'NONE',  ( 9.762153702110021092E-27, 46.00000000000018474, -25.00000000000000000 ) ) ;
#9189=ORIENTED_EDGE ( 'NONE', *, *, #2646, .T. ) ;
#9190=CIRCLE ( 'NONE', #3339, 26.00000000000006395 ) ;
#9204=EDGE_CURVE ( 'NONE', #6709, #3624, #5584, .T. ) ;
#9223=DIRECTION ( 'NONE',  ( -1.735493991486225972E-29, 6.508102468073347395E-30, 1.000000000000000000 ) ) ;
#9225=DIRECTION ( 'NONE',  ( -0.1666666666666658525, -3.897465909857536228E-29, -0.9860132971832695770 ) ) ;
#9226=( NAMED_UNIT ( * ) SI_UNIT ( $, .STERADIAN. ) SOLID_ANGLE_UNIT ( ) );
#9241=ORIENTED_EDGE ( 'NONE', *, *, #649, .F. ) ;
#9252=VECTOR ( 'NONE', #260, 1000.000000000000000 ) ;
#9265=AXIS2_PLACEMENT_3D ( 'NONE', #9612, #8781, #7290 ) ;
#9274=FACE_OUTER_BOUND ( 'NONE', #7094, .T. ) ;
#9278=EDGE_CURVE ( 'NONE', #8311, #7524, #2194, .T. ) ;
#9279=CARTESIAN_POINT ( 'NONE',  ( -8.216777476527294510, 52.00000000000031974, -23.61111111111111427 ) ) ;
#9281=DIRECTION ( 'NONE',  ( -1.820952055660014662E-28, -1.000000000000000000, -7.038118388768679669E-30 ) ) ;
#9286=ORIENTED_EDGE ( 'NONE', *, *, #7837, .F. ) ;
#9293=ORIENTED_EDGE ( 'NONE', *, *, #1489, .T. ) ;
#9294=DIRECTION ( 'NONE',  ( 0.9860132971832693549, 1.788557213313974126E-28, -0.1666666666666657970 ) ) ;
#9318=DIRECTION ( 'NONE',  ( -1.820952055660014662E-28, -1.000000000000000000, -7.038118388768679669E-30 ) ) ;
#9319=MECHANICAL_DESIGN_GEOMETRIC_PRESENTATION_REPRESENTATION('',(#5848),#6781);
#9322=CARTESIAN_POINT ( 'NONE',  ( 1.203012880462043003E-26, 59.00000000000029843, -37.00000000000000711 ) ) ;
#9342=CARTESIAN_POINT ( 'NONE',  ( -8.216777476527294510, 44.50000000000019185, -23.61111111111111427 ) ) ;
#9345=VECTOR ( 'NONE', #3951, 1000.000000000000000 ) ;
#9348=EDGE_LOOP ( 'NONE', ( #959, #4993, #6210, #8098 ) ) ;
#9354=VECTOR ( 'NONE', #9575, 1000.000000000000000 ) ;
#9356=LINE ( 'NONE', #6384, #3998 ) ;
#9361=DIRECTION ( 'NONE',  ( -1.820952055660014662E-28, -1.000000000000000000, -7.038118388768679669E-30 ) ) ;
#9366=CARTESIAN_POINT ( 'NONE',  ( -8.545448575588375562, -1.756255516286720374E-27, -24.55555555555558911 ) ) ;
#9390=EDGE_CURVE ( 'NONE', #3249, #7030, #1679, .T. ) ;
#9391=VERTEX_POINT ( 'NONE', #4700 ) ;
#9393=AXIS2_PLACEMENT_3D ( 'NONE', #6009, #1683, #9043 ) ;
#9395=CARTESIAN_POINT ( 'NONE',  ( 8.677469957431129860E-27, 45.50000000000019185, -24.09806918451535651 ) ) ;
#9397=AXIS2_PLACEMENT_3D ( 'NONE', #83, #6135, #6093 ) ;
#9408=AXIS2_PLACEMENT_3D ( 'NONE', #701, #854, #3054 ) ;
#9412=PLANE ( 'NONE',  #5610 ) ;
#9424=FACE_OUTER_BOUND ( 'NONE', #1056, .T. ) ;
#9428=VERTEX_POINT ( 'NONE', #9433 ) ;
#9433=CARTESIAN_POINT ( 'NONE',  ( -8.545448575588393325, 50.50000000000031974, -24.55555555555563529 ) ) ;
#9434=ORIENTED_EDGE ( 'NONE', *, *, #7997, .F. ) ;
#9442=EDGE_CURVE ( 'NONE', #6031, #7876, #9523, .T. ) ;
#9447=ADVANCED_FACE ( 'NONE', ( #2794 ), #8690, .F. ) ;
#9451=ORIENTED_EDGE ( 'NONE', *, *, #8819, .F. ) ;
#9452=CARTESIAN_POINT ( 'NONE',  ( 1.084683744678891232E-26, 53.50000000000031264, -25.00000000000000000 ) ) ;
#9453=ORIENTED_EDGE ( 'NONE', *, *, #1898, .F. ) ;
#9460=EDGE_CURVE ( 'NONE', #77, #2117, #4882, .T. ) ;
#9462=VECTOR ( 'NONE', #3527, 1000.000000000000000 ) ;
#9466=DIRECTION ( 'NONE',  ( 1.735493991486224571E-29, 0.000000000000000000, -1.000000000000000000 ) ) ;
#9472=ORIENTED_EDGE ( 'NONE', *, *, #8073, .F. ) ;
#9476=LINE ( 'NONE', #6638, #9354 ) ;
#9484=EDGE_LOOP ( 'NONE', ( #1859, #6769, #8711, #8416 ) ) ;
#9499=LINE ( 'NONE', #5555, #8566 ) ;
#9509=ADVANCED_FACE ( 'NONE', ( #4345 ), #1178, .F. ) ;
#9511=CARTESIAN_POINT ( 'NONE',  ( 5.423418723394456162E-28, -2.066522830327504070E-28, -26.00000000000015987 ) ) ;
#9522=CARTESIAN_POINT ( 'NONE',  ( -8.216777476527274970, 47.00000000000034106, -23.61111111111107519 ) ) ;
#9523=LINE ( 'NONE', #1230, #7519 ) ;
#9524=ADVANCED_FACE ( 'NONE', ( #6499 ), #9576, .F. ) ;
#9528=CIRCLE ( 'NONE', #1015, 26.00000000000006395 ) ;
#9542=FACE_OUTER_BOUND ( 'NONE', #2504, .T. ) ;
#9545=ORIENTED_EDGE ( 'NONE', *, *, #4693, .F. ) ;
#9546=ORIENTED_EDGE ( 'NONE', *, *, #3777, .T. ) ;
#9547=LINE ( 'NONE', #2029, #8436 ) ;
#9561=DIRECTION ( 'NONE',  ( 1.735493991486224571E-29, 0.000000000000000000, -1.000000000000000000 ) ) ;
#9566=EDGE_CURVE ( 'NONE', #3257, #2396, #4540, .T. ) ;
#9573=EDGE_CURVE ( 'NONE', #2848, #2873, #125, .T. ) ;
#9575=DIRECTION ( 'NONE',  ( 1.735493991486225972E-29, -6.508102468073347395E-30, -1.000000000000000000 ) ) ;
#9576=PLANE ( 'NONE',  #3901 ) ;
#9579=ADVANCED_FACE ( 'NONE', ( #3688 ), #6836, .F. ) ;
#9582=EDGE_CURVE ( 'NONE', #8853, #9115, #6042, .T. ) ;
#9587=VERTEX_POINT ( 'NONE', #8932 ) ;
#9606=DIRECTION ( 'NONE',  ( -1.735493991486225972E-29, 6.508102468073347395E-30, 1.000000000000000000 ) ) ;
#9611=VERTEX_POINT ( 'NONE', #2942 ) ;
#9612=CARTESIAN_POINT ( 'NONE',  ( 7.742466688136331219E-27, 42.50000000000020606, 2.935117235246147440E-28 ) ) ;
#9615=FACE_OUTER_BOUND ( 'NONE', #7820, .T. ) ;
#9616=CARTESIAN_POINT ( 'NONE',  ( 8.283039504820623957E-27, 44.50000000000019185, -24.09806918451535651 ) ) ;
#9622=VERTEX_POINT ( 'NONE', #3034 ) ;
#9625=ORIENTED_EDGE ( 'NONE', *, *, #7146, .T. ) ;
#9626=ADVANCED_FACE ( 'NONE', ( #8335 ), #4436, .F. ) ;
#9628=AXIS2_PLACEMENT_3D ( 'NONE', #3677, #3731, #9561 ) ;
#9630=LINE ( 'NONE', #7307, #8553 ) ;
#9640=LINE ( 'NONE', #4411, #7190 ) ;
#9646=DIRECTION ( 'NONE',  ( -0.9860132971832693549, -1.788557213313974126E-28, 0.1666666666666657970 ) ) ;
#9647=MANIFOLD_SOLID_BREP ( 'Chamfer2', #6088 ) ;
#9653=DIRECTION ( 'NONE',  ( 1.735493991486225972E-29, -6.508102468073347395E-30, -1.000000000000000000 ) ) ;
#9654=CARTESIAN_POINT ( 'NONE',  ( 0.000000000000000000, 0.000000000000000000, 0.000000000000000000 ) ) ;
#9658=ADVANCED_FACE ( 'NONE', ( #9274 ), #9027, .F. ) ;
#9661=CARTESIAN_POINT ( 'NONE',  ( 1.040310318760209318E-26, 50.00000000000032685, -25.00000000000000000 ) ) ;
#9663=DIRECTION ( 'NONE',  ( -1.820952055660014662E-28, -1.000000000000000000, -7.038118388768679669E-30 ) ) ;
#9669=DIRECTION ( 'NONE',  ( -0.9860132971832694659, -1.788557213313974350E-28, 0.1666666666666658247 ) ) ;
#9671=ORIENTED_EDGE ( 'NONE', *, *, #7093, .T. ) ;
#9672=CARTESIAN_POINT ( 'NONE',  ( 1.084683744678891232E-26, 53.00000000000031974, -25.00000000000000000 ) ) ;
#9702=ORIENTED_EDGE ( 'NONE', *, *, #3287, .F. ) ;
#9706=VECTOR ( 'NONE', #6984, 1000.000000000000000 ) ;
#9708=DIRECTION ( 'NONE',  ( 1.820952055660014662E-28, 1.000000000000000000, -6.508102468073347395E-30 ) ) ;
#9719=AXIS2_PLACEMENT_3D ( 'NONE', #70, #9053, #3010 ) ;
#9727=CARTESIAN_POINT ( 'NONE',  ( -8.216777476527294510, 54.50000000000031264, -23.61111111111111427 ) ) ;
#9729=ORIENTED_EDGE ( 'NONE', *, *, #3351, .T. ) ;
#9731=CIRCLE ( 'NONE', #9265, 26.00000000000017408 ) ;
#9733=ORIENTED_EDGE ( 'NONE', *, *, #760, .F. ) ;
#9740=VERTEX_POINT ( 'NONE', #1120 ) ;
#9742=VERTEX_POINT ( 'NONE', #4138 ) ;
#9753=CARTESIAN_POINT ( 'NONE',  ( -8.216777476527294510, 45.50000000000019185, -23.61111111111111427 ) ) ;
#9800=COLOUR_RGB('Off White',0.89,0.88,0.83);
#9801=FILL_AREA_STYLE_COLOUR('',#9800);
#9802=FILL_AREA_STYLE('',(#9801));
#9803=SURFACE_STYLE_FILL_AREA(#9802);
#9804=SURFACE_SIDE_STYLE('',(#9803));
#9805=SURFACE_STYLE_USAGE(.BOTH.,#9804);
#9806=PRESENTATION_STYLE_ASSIGNMENT((#9805));
ENDSEC;
END-ISO-10303-21;
